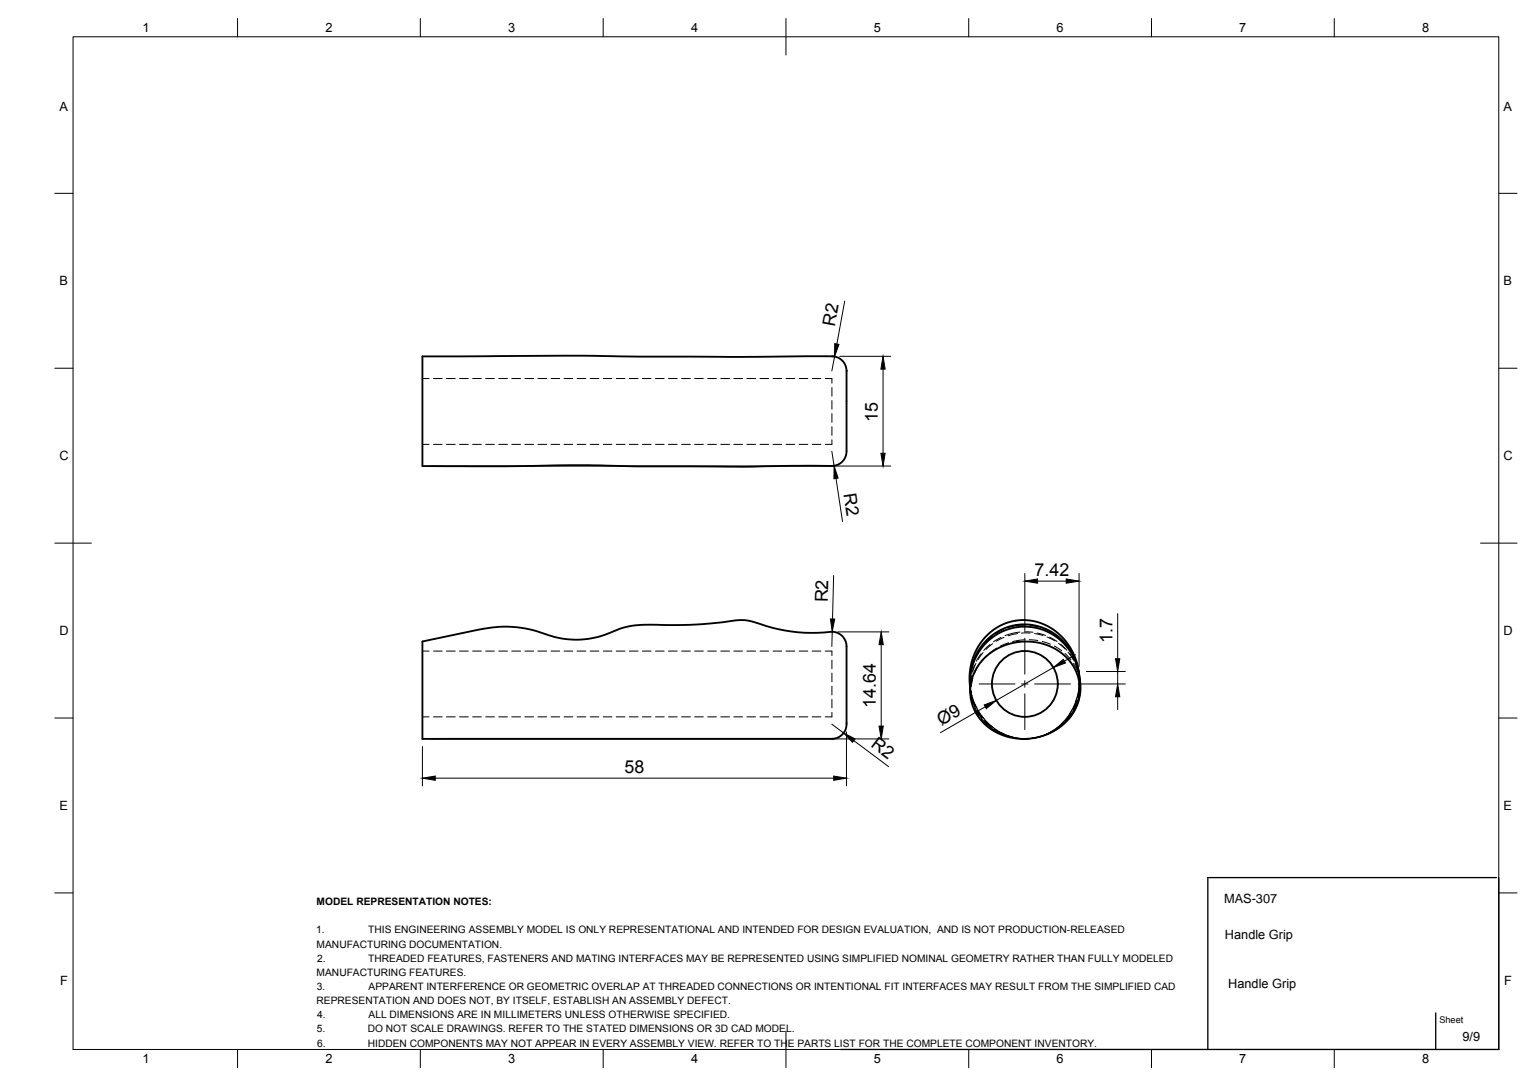
ISO-10303-21;
HEADER;
FILE_DESCRIPTION (('STEP AP214'),
    '1' );
FILE_NAME ('Handle Grip.step',
    '2026-10-06T07:34:29',
    ( '' ),
    ( '' ),
    'SwSTEP 2.0',
    'SolidWorks 2025',
    '' );
FILE_SCHEMA (( 'AUTOMOTIVE_DESIGN' ));
ENDSEC;

DATA;
#6=CARTESIAN_POINT ( 'NONE',  ( -167.5053995445195767, 127.4304153265770907, 2.500000001036336350 ) ) ;
#10=CARTESIAN_POINT ( 'NONE',  ( -168.3602667112202766, 125.8948777600411830, -3.002243219525047024 ) ) ;
#25=CARTESIAN_POINT ( 'NONE',  ( -225.5636091402884915, 143.1065995042388863, -0.5218507872395625746 ) ) ;
#28=CARTESIAN_POINT ( 'NONE',  ( -185.2335129678179726, 125.0353967269121966, 9.577123744044223841 ) ) ;
#58=FACE_OUTER_BOUND ( 'NONE', #1129, .T. ) ;
#68=CARTESIAN_POINT ( 'NONE',  ( -223.5763732829059904, 146.6670444861485976, 6.843617190574383891 ) ) ;
#87=CARTESIAN_POINT ( 'NONE',  ( -207.0700983879231387, 149.0508413170868209, -0.4547266291960758156 ) ) ;
#99=CARTESIAN_POINT ( 'NONE',  ( -218.1518098834511648, 139.2461763302102327, 3.478895870929506362 ) ) ;
#102=CARTESIAN_POINT ( 'NONE',  ( -182.6699909761611877, 123.4132960977408970, 9.577123744044220288 ) ) ;
#112=CARTESIAN_POINT ( 'NONE',  ( -225.3482675701515348, 143.4924177300907502, -0.7821592797845021705 ) ) ;
#133=CARTESIAN_POINT ( 'NONE',  ( -221.9693044472552117, 149.5463605724702916, 7.947916423171728084 ) ) ;
#136=CARTESIAN_POINT ( 'NONE',  ( -222.7380986314676363, 148.1689451111236906, 7.733218891984481758 ) ) ;
#137=EDGE_CURVE ( 'NONE', #9526, #14472, #1038, .T. ) ;
#142=CIRCLE ( 'NONE', #13010, 4.499999999999950262 ) ;
#146=B_SPLINE_CURVE_WITH_KNOTS ( 'NONE', 3,
 ( #5136, #531, #1653, #11218, #9963, #14979, #8698, #12464, #14906, #1729, #5371, #4019, #13643, #371, #7438, #2772, #5212, #6490, #11287, #14749, #7674, #6569, #448, #13727, #10034, #10112, #10189, #12233, #8933, #1411, #2930, #11372, #4170, #6248, #1492, #211, #11061, #2692, #5059, #9884, #14674, #3874, #685, #1881, #15369, #849, #13889, #9240 ),
 .UNSPECIFIED., .F., .F.,
 ( 4, 2, 2, 2, 2, 2, 2, 2, 2, 2, 2, 2, 2, 2, 2, 2, 2, 2, 2, 2, 2, 2, 2, 4 ),
 ( 0.02192817935270313656, 0.02330785662426448565, 0.02399769526004516540, 0.02468753389582584862, 0.02606721116738722893, 0.02675704980316793297, 0.02744688843894863700, 0.02882656571051007630, 0.02951640434629079768, 0.03020624298207151559, 0.03158592025363299305, 0.03227575888941371096, 0.03296559752519442887, 0.03365543616097514679, 0.03434527479675586470, 0.03572495206831733522, 0.03641479070409808783, 0.03710462933987884043, 0.03779446797565959304, 0.03848430661144034565, 0.03986398388300183004, 0.04124366115456330750, 0.04262333842612478496, 0.04400301569768626936 ),
 .UNSPECIFIED. ) ;
#156=CARTESIAN_POINT ( 'NONE',  ( -179.9223906590855222, 134.3711564447467310, 1.515441477536284554 ) ) ;
#157=CARTESIAN_POINT ( 'NONE',  ( -223.6137413416247739, 142.0138547493179146, 2.263321283727593336 ) ) ;
#159=CIRCLE ( 'NONE', #9018, 4.499999999999950262 ) ;
#170=CARTESIAN_POINT ( 'NONE',  ( -183.7136537759689929, 127.7093858820786068, -5.230826428279597096 ) ) ;
#173=CARTESIAN_POINT ( 'NONE',  ( -197.4591130885309553, 135.0981391493542105, 10.16010209732750802 ) ) ;
#189=ORIENTED_EDGE ( 'NONE', *, *, #8600, .F. ) ;
#199=CARTESIAN_POINT ( 'NONE',  ( -185.2055264765504887, 137.3096093875189467, 2.500000000000000000 ) ) ;
#206=CARTESIAN_POINT ( 'NONE',  ( -224.5476011597490356, 144.9269372877251669, 3.604463283145519448 ) ) ;
#209=CARTESIAN_POINT ( 'NONE',  ( -222.3356595723642215, 144.5667354790973604, 8.419022500423421818 ) ) ;
#211=CARTESIAN_POINT ( 'NONE',  ( -172.9645346626803359, 118.3395572346633173, -3.768257758897336274 ) ) ;
#254=CARTESIAN_POINT ( 'NONE',  ( -176.4863952559862526, 117.0241230567913959, -0.6469977504890583875 ) ) ;
#257=CARTESIAN_POINT ( 'NONE',  ( -171.9895241055258168, 125.0924944214600885, 9.516496325551347724 ) ) ;
#271=CARTESIAN_POINT ( 'NONE',  ( -218.6464950597879238, 155.4996951832063701, 5.432615396193927637 ) ) ;
#288=CARTESIAN_POINT ( 'NONE',  ( -167.5097532647548633, 127.4226149533560175, 3.478855110549762042 ) ) ;
#292=CARTESIAN_POINT ( 'NONE',  ( -221.1247960154559280, 151.0594299935001743, 7.622044586438916802 ) ) ;
#294=CARTESIAN_POINT ( 'NONE',  ( -220.5689849208904150, 152.0552528170083519, 9.261189829759533865 ) ) ;
#304=B_SPLINE_CURVE_WITH_KNOTS ( 'NONE', 3,
 ( #12178, #157, #5002, #3249, #8007 ),
 .UNSPECIFIED., .F., .F.,
 ( 4, 1, 4 ),
 ( 2.671544684753287039E-05, 0.0004182544953931666577, 0.0008097935439387997673 ),
 .UNSPECIFIED. ) ;
#316=CARTESIAN_POINT ( 'NONE',  ( -214.8715905313398480, 153.8675021612092451, 2.500000000000000000 ) ) ;
#328=CARTESIAN_POINT ( 'NONE',  ( -223.3178949021943538, 142.5860305806809833, -0.6404123112780930605 ) ) ;
#330=CARTESIAN_POINT ( 'NONE',  ( -207.1238489746795608, 137.1336079999123854, -4.642206099735007641 ) ) ;
#333=CARTESIAN_POINT ( 'NONE',  ( -199.4124801547868913, 127.6177204676982910, 1.515400478619089109 ) ) ;
#358=CARTESIAN_POINT ( 'NONE',  ( -218.4414990732828699, 155.8669776719573861, 2.805362964459314323 ) ) ;
#359=CARTESIAN_POINT ( 'NONE',  ( -218.6464950597879238, 155.4996951832063701, 5.432615396193927637 ) ) ;
#367=CARTESIAN_POINT ( 'NONE',  ( -220.9628981692495699, 151.3494953986536018, 7.483278023344910324 ) ) ;
#369=CARTESIAN_POINT ( 'NONE',  ( -219.7507648086670429, 149.4749995001899663, 9.873895959572530856 ) ) ;
#371=CARTESIAN_POINT ( 'NONE',  ( -168.7841562197520489, 125.8293614238909299, -3.029850393553606303 ) ) ;
#395=CARTESIAN_POINT ( 'NONE',  ( -187.5347606140533969, 120.9941390333424636, 2.431555724346869063 ) ) ;
#405=CARTESIAN_POINT ( 'NONE',  ( -217.9852252332578928, 152.6415593000486126, -3.308226381094188095 ) ) ;
#406=CARTESIAN_POINT ( 'NONE',  ( -195.7742941377835280, 134.4381891934308442, -5.230826428279600648 ) ) ;
#409=CARTESIAN_POINT ( 'NONE',  ( -199.2256335332332640, 127.9713659812714042, 5.434137442415931218 ) ) ;
#443=CARTESIAN_POINT ( 'NONE',  ( -224.5811800873043182, 144.8667753680073531, 1.831365460742872209 ) ) ;
#446=CARTESIAN_POINT ( 'NONE',  ( -218.2326813014511799, 152.2161514369302324, 8.572300711411607210 ) ) ;
#448=CARTESIAN_POINT ( 'NONE',  ( -170.5205985377005220, 122.7182524358224640, -5.056862372992222632 ) ) ;
#483=CARTESIAN_POINT ( 'NONE',  ( -221.4307639069678544, 146.2562371466928255, -4.592498632207916209 ) ) ;
#485=CARTESIAN_POINT ( 'NONE',  ( -176.9844935205031504, 127.5518652045528825, -4.662307221713766658 ) ) ;
#488=CARTESIAN_POINT ( 'NONE',  ( -173.0737465816261818, 117.4314230949052558, 7.694953281110847421 ) ) ;
#500=CARTESIAN_POINT ( 'NONE',  ( -198.5721217036497990, 144.7598446228703324, 3.478855109513426580 ) ) ;
#517=CARTESIAN_POINT ( 'NONE',  ( -219.4169908596040273, 154.1192310103966179, 2.706804888356528771 ) ) ;
#529=CARTESIAN_POINT ( 'NONE',  ( -219.5915661803683463, 153.8064519195449407, 4.439938623566930254 ) ) ;
#531=CARTESIAN_POINT ( 'NONE',  ( -167.7969933075935387, 127.5980187394608549, 2.035704077629012954 ) ) ;
#543=MECHANICAL_DESIGN_GEOMETRIC_PRESENTATION_REPRESENTATION('',(#10911),#10658);
#570=CARTESIAN_POINT ( 'NONE',  ( -202.8891874331996519, 144.7632710727894505, -2.963320117457099112 ) ) ;
#573=CARTESIAN_POINT ( 'NONE',  ( -186.4931015233695462, 122.8215886266871593, 7.918248976830652097 ) ) ;
#586=CARTESIAN_POINT ( 'NONE',  ( -182.6699909761611877, 123.4132960977408970, 9.577123744044220288 ) ) ;
#599=CARTESIAN_POINT ( 'NONE',  ( -169.3917585582371714, 124.7407464570165700, 8.854531459401838944 ) ) ;
#600=CARTESIAN_POINT ( 'NONE',  ( -219.0516113763855799, 154.7738657095153769, -1.749095451262919765 ) ) ;
#611=CARTESIAN_POINT ( 'NONE',  ( -220.4620190166787950, 152.2468990252863819, 9.155722436418765042 ) ) ;
#647=CARTESIAN_POINT ( 'NONE',  ( -187.0868153883506011, 133.8486679469899343, -4.640918829492425957 ) ) ;
#650=CARTESIAN_POINT ( 'NONE',  ( -214.6174474432871762, 135.6318802667844921, 5.434137442415934771 ) ) ;
#661=CARTESIAN_POINT ( 'NONE',  ( -191.1905365997726562, 133.0085349363843363, 10.16010209732750624 ) ) ;
#671=CARTESIAN_POINT ( 'NONE',  ( -169.9972604110092789, 123.6558948400181634, 9.476346162107795124 ) ) ;
#672=CARTESIAN_POINT ( 'NONE',  ( -218.9426345149119300, 150.9185095621452035, -4.524781484457172986 ) ) ;
#685=CARTESIAN_POINT ( 'NONE',  ( -173.9738588760758944, 116.5311944691898560, -0.9961046041182962663 ) ) ;
#700=CARTESIAN_POINT ( 'NONE',  ( -225.6985468192879409, 142.8648374703979016, 2.076118051499458161 ) ) ;
#713=APPLICATION_CONTEXT ( 'automotive_design' ) ;
#717=ADVANCED_FACE ( 'NONE', ( #1332, #7434 ), #1486, .F. ) ;
#722=CARTESIAN_POINT ( 'NONE',  ( -169.4320859569187405, 123.9702250307836238, -4.722862203412457660 ) ) ;
#725=CARTESIAN_POINT ( 'NONE',  ( -195.7742941377835280, 134.4381891934308442, -5.230826428279600648 ) ) ;
#742=CARTESIAN_POINT ( 'NONE',  ( -174.5069932933876942, 126.2863744793834826, 9.536681319450917016 ) ) ;
#756=CARTESIAN_POINT ( 'NONE',  ( -173.9115424460105430, 116.6428441356814432, 5.774694861875956597 ) ) ;
#757=CARTESIAN_POINT ( 'NONE',  ( -222.4281468042453298, 148.7242724638446703, -5.036090039102246507 ) ) ;
#765=EDGE_CURVE ( 'NONE', #9030, #14554, #2287, .T. ) ;
#766=CARTESIAN_POINT ( 'NONE',  ( -219.7707515679132655, 153.4854131703968392, -0.3598758019112536233 ) ) ;
#773=CARTESIAN_POINT ( 'NONE',  ( -170.1275826011421941, 128.8939672761866859, 2.500000000760459695 ) ) ;
#805=CARTESIAN_POINT ( 'NONE',  ( -170.8299300849453459, 127.1729693371208043, -2.992655347556774981 ) ) ;
#808=CARTESIAN_POINT ( 'NONE',  ( -219.6417540138374704, 145.3326194796887023, -4.642206099735023628 ) ) ;
#824=CARTESIAN_POINT ( 'NONE',  ( -216.9711578880983893, 150.1110767499728240, 9.578254705571840333 ) ) ;
#835=CARTESIAN_POINT ( 'NONE',  ( -168.4340493060770427, 126.4566329172550070, 6.894248570768724882 ) ) ;
#836=CARTESIAN_POINT ( 'NONE',  ( -222.5645123348796801, 148.4799522099133640, -2.927675643679180428 ) ) ;
#849=CARTESIAN_POINT ( 'NONE',  ( -174.2601771783465097, 116.0182102862799383, 1.243088744850515459 ) ) ;
#850=CARTESIAN_POINT ( 'NONE',  ( -216.7144175016715337, 154.8588128942135143, 3.150775860475527601 ) ) ;
#853=CARTESIAN_POINT ( 'NONE',  ( -210.7165899865938172, 151.5484195431892545, 2.500000000000000000 ) ) ;
#859=EDGE_CURVE ( 'NONE', #14554, #9030, #3433, .T. ) ;
#867=CARTESIAN_POINT ( 'NONE',  ( -223.5869895076567957, 142.0744606454175312, 3.511683908622253991 ) ) ;
#886=CARTESIAN_POINT ( 'NONE',  ( -191.3370974917540366, 126.0439545877573266, -0.4555467707853441128 ) ) ;
#897=SURFACE_STYLE_FILL_AREA ( #8426 ) ;
#901=CARTESIAN_POINT ( 'NONE',  ( -185.2335129678179726, 125.0353967269121966, 9.577123744044223841 ) ) ;
#914=CARTESIAN_POINT ( 'NONE',  ( -221.3664521364747202, 150.6264651190829511, -2.887957967080375443 ) ) ;
#964=CARTESIAN_POINT ( 'NONE',  ( -223.5232045190763301, 146.7623046726374980, -4.689260562946596878 ) ) ;
#978=CARTESIAN_POINT ( 'NONE',  ( -214.6152097961127367, 135.6358893629490581, -0.4555467707853336767 ) ) ;
#992=CARTESIAN_POINT ( 'NONE',  ( -222.3946175953714999, 148.7843453047176467, -2.994737441843033476 ) ) ;
#1000=CARTESIAN_POINT ( 'NONE',  ( -206.0179204244930702, 148.9258921110169638, 2.500000000000000000 ) ) ;
#1007=AXIS2_PLACEMENT_3D ( 'NONE', #2898, #5252, #7561 ) ;
#1011=CARTESIAN_POINT ( 'NONE',  ( -216.7032046242510148, 154.8780296845847033, 2.891444798692482721 ) ) ;
#1013=CARTESIAN_POINT ( 'NONE',  ( -193.7200834347810599, 142.0619459586758921, 2.500000000000000000 ) ) ;
#1038=CIRCLE ( 'NONE', #11412, 4.499999999999950262 ) ;
#1051=CARTESIAN_POINT ( 'NONE',  ( -181.1480734112017501, 126.1383063644306617, -5.230826428279600648 ) ) ;
#1053=EDGE_LOOP ( 'NONE', ( #1556, #9864 ) ) ;
#1066=CARTESIAN_POINT ( 'NONE',  ( -213.9961813491638623, 134.6717504882919911, 1.515400478619087776 ) ) ;
#1073=CARTESIAN_POINT ( 'NONE',  ( -217.6653619995784652, 138.6635820529667740, 2.431555724346871283 ) ) ;
#1078=CARTESIAN_POINT ( 'NONE',  ( -219.3877568461323619, 150.1024971847152756, -4.823803736792959818 ) ) ;
#1079=CARTESIAN_POINT ( 'NONE',  ( -223.4717893243274602, 142.3106348291761662, 4.713848895078025514 ) ) ;
#1089=ORIENTED_EDGE ( 'NONE', *, *, #5398, .F. ) ;
#1094=CARTESIAN_POINT ( 'NONE',  ( -218.4488137430494419, 155.8538722928748541, 3.478855109783925315 ) ) ;
#1105=CARTESIAN_POINT ( 'NONE',  ( -224.7518895393548348, 144.5609225879004498, 7.521475632127809341 ) ) ;
#1111=CYLINDRICAL_SURFACE ( 'NONE', #6828, 4.499999999999950262 ) ;
#1127=CARTESIAN_POINT ( 'NONE',  ( -216.9311889273521672, 150.1826874172201656, -4.640918829492440167 ) ) ;
#1129=EDGE_LOOP ( 'NONE', ( #6452, #6459, #7636, #5771, #1089 ) ) ;
#1140=CARTESIAN_POINT ( 'NONE',  ( -225.7548303624724610, 142.7639966680278576, 1.446957622915672204 ) ) ;
#1144=CARTESIAN_POINT ( 'NONE',  ( -203.7296541848517109, 135.3294987143146955, 9.577123744044227394 ) ) ;
#1155=CARTESIAN_POINT ( 'NONE',  ( -218.9545055651059045, 150.9247396209540568, 9.391049919365073606 ) ) ;
#1176=CARTESIAN_POINT ( 'NONE',  ( -224.5448265106511769, 144.9319085071302879, 3.590746859383691536 ) ) ;
#1194=CARTESIAN_POINT ( 'NONE',  ( -202.8891874331996519, 144.7632710727894505, -2.963320117457099112 ) ) ;
#1212=CARTESIAN_POINT ( 'NONE',  ( -191.4964613557999655, 125.7493975051623352, 3.478895870929489043 ) ) ;
#1215=CARTESIAN_POINT ( 'NONE',  ( -210.0240857098682454, 141.7683007401625446, 10.16010209732750624 ) ) ;
#1228=CARTESIAN_POINT ( 'NONE',  ( -224.5811800873044604, 144.8667753680074384, 1.831365460742872209 ) ) ;
#1258=CARTESIAN_POINT ( 'NONE',  ( -221.2417723974670878, 146.6801937162670697, 9.651042165284529517 ) ) ;
#1280=CARTESIAN_POINT ( 'NONE',  ( -178.3861577417919477, 131.0834419243807076, -2.963320117457100888 ) ) ;
#1295=CARTESIAN_POINT ( 'NONE',  ( -200.9709139173866959, 128.5579952147370761, 5.434137442415933883 ) ) ;
#1298=CARTESIAN_POINT ( 'NONE',  ( -216.9711578880983893, 150.1110767499728240, 9.578254705571840333 ) ) ;
#1308=CARTESIAN_POINT ( 'NONE',  ( -225.6439726407676005, 142.9626156777225390, 1.090105839479173833 ) ) ;
#1316=CARTESIAN_POINT ( 'NONE',  ( -198.5677679834141713, 144.7676449960911498, 2.500000000000000000 ) ) ;
#1332=FACE_BOUND ( 'NONE', #3235, .T. ) ;
#1335=CARTESIAN_POINT ( 'NONE',  ( -224.2877105866247973, 145.3925720454151929, 5.086385912607861215 ) ) ;
#1342=CARTESIAN_POINT ( 'NONE',  ( -220.3531759299249302, 148.3382346779569616, 2.431557144026069928 ) ) ;
#1355=CARTESIAN_POINT ( 'NONE',  ( -188.7806045336324132, 137.2844789098840863, -2.963320117457101777 ) ) ;
#1369=CARTESIAN_POINT ( 'NONE',  ( -216.7159361415700403, 154.8568568287998630, 1.560284994380096046 ) ) ;
#1370=CARTESIAN_POINT ( 'NONE',  ( -183.9200705329474772, 121.1751083001002485, -2.964974570226829087 ) ) ;
#1373=CARTESIAN_POINT ( 'NONE',  ( -212.4168668197547731, 139.5435760318306677, 9.577123744044230946 ) ) ;
#1378=EDGE_CURVE ( 'NONE', #4070, #14472, #12986, .T. ) ;
#1385=CARTESIAN_POINT ( 'NONE',  ( -169.9361637590235716, 128.7768979049109532, 3.478855110294483133 ) ) ;
#1407=CARTESIAN_POINT ( 'NONE',  ( -221.6235305807591658, 150.1658687316387670, 7.893372954062758851 ) ) ;
#1409=CARTESIAN_POINT ( 'NONE',  ( -224.3998921539632931, 145.1915811579927151, 4.610672262717653069 ) ) ;
#1411=CARTESIAN_POINT ( 'NONE',  ( -171.8695707977107645, 120.3013568790891554, -4.955367435459418601 ) ) ;
#1432=CARTESIAN_POINT ( 'NONE',  ( -195.9617019660094570, 137.8802668252396586, -4.640918829492428621 ) ) ;
#1442=CARTESIAN_POINT ( 'NONE',  ( -217.5100339609262221, 153.4805093641580527, -2.286312808770087912 ) ) ;
#1444=CARTESIAN_POINT ( 'NONE',  ( -205.6342130761154863, 139.8173426991758959, -5.230826428279590878 ) ) ;
#1448=CARTESIAN_POINT ( 'NONE',  ( -181.1823003367078115, 126.0769834546670296, 10.16010209732750624 ) ) ;
#1451=ORIENTED_EDGE ( 'NONE', *, *, #9650, .T. ) ;
#1460=CARTESIAN_POINT ( 'NONE',  ( -186.0759242617834559, 135.7072545306847076, 7.919662025281895446 ) ) ;
#1477=CARTESIAN_POINT ( 'NONE',  ( -206.2408270422487249, 148.5277750773568926, 5.434754235172608361 ) ) ;
#1486=PLANE ( 'NONE',  #8630 ) ;
#1490=CARTESIAN_POINT ( 'NONE',  ( -219.4551987602064855, 154.0507755588392911, 3.411546396426036409 ) ) ;
#1492=CARTESIAN_POINT ( 'NONE',  ( -172.7841977562675311, 118.6626591106209787, -4.047107877712195823 ) ) ;
#1530=CARTESIAN_POINT ( 'NONE',  ( -220.2566479300740241, 148.4875731452288221, -5.069746451151177169 ) ) ;
#1531=CARTESIAN_POINT ( 'NONE',  ( -212.3935931674892856, 139.5852744332111683, -4.642206099735020963 ) ) ;
#1534=CARTESIAN_POINT ( 'NONE',  ( -217.9748787080196450, 139.5740753954225966, -0.4555467707853197989 ) ) ;
#1549=CARTESIAN_POINT ( 'NONE',  ( -218.4488137430494419, 155.8538722928748541, 3.478855109783925315 ) ) ;
#1556=ORIENTED_EDGE ( 'NONE', *, *, #3132, .T. ) ;
#1564=CARTESIAN_POINT ( 'NONE',  ( -185.3757041553864156, 136.9956776582455973, 5.434754235172603920 ) ) ;
#1571=CARTESIAN_POINT ( 'NONE',  ( -221.8318359980363539, 149.7926568781921048, 9.921711862944807336 ) ) ;
#1594=CARTESIAN_POINT ( 'NONE',  ( -169.9274309510963406, 128.7925441011331031, 1.515441478317341994 ) ) ;
#1612=CARTESIAN_POINT ( 'NONE',  ( -216.6980668629938123, 154.8869363267023687, 2.500000000158653091 ) ) ;
#1614=CARTESIAN_POINT ( 'NONE',  ( -202.2493014528935475, 138.0335512477381883, -5.230826428279597096 ) ) ;
#1617=CARTESIAN_POINT ( 'NONE',  ( -194.2694872093395873, 127.5478817636406035, 5.434137442415935659 ) ) ;
#1629=CARTESIAN_POINT ( 'NONE',  ( -169.2610106913410277, 124.9750017845142764, 2.431557144026069928 ) ) ;
#1643=CARTESIAN_POINT ( 'NONE',  ( -207.0940556909077657, 149.0079180481279479, 5.434754235172608361 ) ) ;
#1649=CARTESIAN_POINT ( 'NONE',  ( -224.5619881126438315, 144.9011608032434992, 1.476503984934130598 ) ) ;
#1651=CARTESIAN_POINT ( 'NONE',  ( -220.7901307343587689, 151.6590353782033560, 9.451677507526856203 ) ) ;
#1653=CARTESIAN_POINT ( 'NONE',  ( -167.8131253141077650, 127.5691157174926644, 1.575245659892765326 ) ) ;
#1686=CARTESIAN_POINT ( 'NONE',  ( -223.4327756907198648, 142.3614043895485963, 0.01469651188060598634 ) ) ;
#1687=CARTESIAN_POINT ( 'NONE',  ( -182.6467173238959560, 123.4549944991208292, -4.642206099735001423 ) ) ;
#1690=CARTESIAN_POINT ( 'NONE',  ( -194.4337897068680547, 127.2572260587109554, 3.478895870929501033 ) ) ;
#1716=CARTESIAN_POINT ( 'NONE',  ( -219.5038107907490144, 153.9636794753398874, -2.869066018171615884 ) ) ;
#1721=PRODUCT_DEFINITION_FORMATION_WITH_SPECIFIED_SOURCE ( 'ANY', '', #8040, .NOT_KNOWN. ) ;
#1725=CARTESIAN_POINT ( 'NONE',  ( -223.5023877966752366, 146.7996010984935538, -2.058674290867560153 ) ) ;
#1727=CARTESIAN_POINT ( 'NONE',  ( -219.7785425680613400, 153.4714543706508891, 5.235913750827374535 ) ) ;
#1729=CARTESIAN_POINT ( 'NONE',  ( -168.3225553318488892, 126.6563918736861325, -1.708925576422542392 ) ) ;
#1731=VERTEX_POINT ( 'NONE', #11313 ) ;
#1767=CARTESIAN_POINT ( 'NONE',  ( -194.3489852843322581, 137.1051365066642234, -4.640918829492427733 ) ) ;
#1770=CARTESIAN_POINT ( 'NONE',  ( -205.9652191273047777, 131.2378527988410326, 1.515400478619091329 ) ) ;
#1782=CARTESIAN_POINT ( 'NONE',  ( -204.9546745879972889, 133.0893851581147374, 7.918248976830629893 ) ) ;
#1793=CARTESIAN_POINT ( 'NONE',  ( -174.2824251065520968, 115.9783496305641535, 2.177446462082195389 ) ) ;
#1794=CARTESIAN_POINT ( 'NONE',  ( -217.7719644788709559, 153.0191138716839134, -2.888063911326615774 ) ) ;
#1806=CARTESIAN_POINT ( 'NONE',  ( -221.2434695521093602, 150.8468077239669753, 9.749916661835451137 ) ) ;
#1840=CARTESIAN_POINT ( 'NONE',  ( -218.4400809351218413, 155.8695184890967482, 1.515441477806783510 ) ) ;
#1843=CARTESIAN_POINT ( 'NONE',  ( -213.9961813491638623, 134.6717504882919911, 1.515400478619087776 ) ) ;
#1856=CARTESIAN_POINT ( 'NONE',  ( -218.3193879687431433, 147.6986783750013217, 10.16010209732750980 ) ) ;
#1868=CARTESIAN_POINT ( 'NONE',  ( -167.8057708040753653, 127.5822924766788447, 2.966601681492425868 ) ) ;
#1869=CARTESIAN_POINT ( 'NONE',  ( -217.8572871788818475, 152.8680898606328356, -3.058345895658412417 ) ) ;
#1881=CARTESIAN_POINT ( 'NONE',  ( -174.1255661870616507, 116.2593870075281473, -0.1232875569927439491 ) ) ;
#1917=CARTESIAN_POINT ( 'NONE',  ( -174.7802519396333878, 131.5011100042426904, 1.515441477806783066 ) ) ;
#1919=ORIENTED_EDGE ( 'NONE', *, *, #7073, .F. ) ;
#1920=CARTESIAN_POINT ( 'NONE',  ( -178.4115273750087738, 119.2860570028907858, -3.078262048313290311 ) ) ;
#1932=CARTESIAN_POINT ( 'NONE',  ( -170.7405378081422214, 121.6209906574826931, 10.02899269843361374 ) ) ;
#1942=CARTESIAN_POINT ( 'NONE',  ( -173.2932605743736474, 117.7505931626010778, 7.695635371731032848 ) ) ;
#1943=CARTESIAN_POINT ( 'NONE',  ( -222.5489981585923545, 148.5077482920355862, -5.007338236124175168 ) ) ;
#1962=ADVANCED_FACE ( 'NONE', ( #8477 ), #1111, .F. ) ;
#1995=CARTESIAN_POINT ( 'NONE',  ( -206.0135413368010404, 148.9337379340180405, 1.515441477536285220 ) ) ;
#1998=CARTESIAN_POINT ( 'NONE',  ( -190.6388552492889517, 127.3288340616119143, -2.964974570226841522 ) ) ;
#2013=CARTESIAN_POINT ( 'NONE',  ( -216.0863581598438543, 143.0557482234525253, 9.577123744044239828 ) ) ;
#2029=CARTESIAN_POINT ( 'NONE',  ( -224.6670067989573454, 144.7130033415326977, -2.813789935910935736 ) ) ;
#2076=CARTESIAN_POINT ( 'NONE',  ( -199.5653198453618700, 142.9393910578133102, -2.963320117457100000 ) ) ;
#2079=CARTESIAN_POINT ( 'NONE',  ( -183.9200705329474772, 121.1751083001002485, -2.964974570226829087 ) ) ;
#2098=CARTESIAN_POINT ( 'NONE',  ( -212.4168668197547731, 139.5435760318306677, 9.577123744044230946 ) ) ;
#2108=CARTESIAN_POINT ( 'NONE',  ( -171.9943068686860386, 120.0778726276766122, 9.490183841837444234 ) ) ;
#2109=CARTESIAN_POINT ( 'NONE',  ( -221.8782673190587786, 149.7094678780528909, -3.059957786404165603 ) ) ;
#2112=CARTESIAN_POINT ( 'NONE',  ( -218.3504703772591711, 152.0071873827878335, 8.737647451593067771 ) ) ;
#2125=CARTESIAN_POINT ( 'NONE',  ( -179.9267697467775520, 134.3633106217456543, 2.500000000000000000 ) ) ;
#2156=CARTESIAN_POINT ( 'NONE',  ( -181.0860728093183809, 120.2032420692993071, -3.023257939496618807 ) ) ;
#2173=CARTESIAN_POINT ( 'NONE',  ( -214.8265656857867327, 135.2606554265309740, 3.478895870929493483 ) ) ;
#2177=CARTESIAN_POINT ( 'NONE',  ( -218.1600191662880661, 152.2676192875508718, 2.431557144026069928 ) ) ;
#2186=CARTESIAN_POINT ( 'NONE',  ( -222.7845331223101084, 143.6298233191951113, -2.509092009812623925 ) ) ;
#2187=CARTESIAN_POINT ( 'NONE',  ( -223.5258475410019230, 142.2005172455266973, 4.260778343889476183 ) ) ;
#2215=FACE_OUTER_BOUND ( 'NONE', #12535, .T. ) ;
#2231=CARTESIAN_POINT ( 'NONE',  ( -167.5010204568278027, 127.4382611495783237, 1.515441478572621570 ) ) ;
#2235=CARTESIAN_POINT ( 'NONE',  ( -183.7136537759689929, 127.7093858820786068, -5.230826428279597096 ) ) ;
#2251=CARTESIAN_POINT ( 'NONE',  ( -175.7482920159357604, 118.3486081613139334, 7.749957389927518925 ) ) ;
#2266=CARTESIAN_POINT ( 'NONE',  ( -225.1194665507443915, 143.9023506720278647, -1.657832751462523291 ) ) ;
#2268=CARTESIAN_POINT ( 'NONE',  ( -222.8945441032406052, 143.4659034320898172, 7.188384078066360594 ) ) ;
#2282=CARTESIAN_POINT ( 'NONE',  ( -185.2055264765504887, 137.3096093875189467, 2.500000000000000000 ) ) ;
#2287=B_SPLINE_CURVE_WITH_KNOTS ( 'NONE', 3,
 ( #9719, #2846, #12229, #14514, #206, #5055, #2688, #11138, #13559, #6405, #11214, #6171, #2763, #14745, #13639, #14817, #3943, #3869, #7668, #133, #9880, #1407, #6240, #292, #367, #14590, #8764, #8694, #6092, #3792, #8614, #13411, #5208, #13484, #14670, #2609, #7590, #7507 ),
 .UNSPECIFIED., .F., .F.,
 ( 4, 2, 2, 2, 2, 2, 2, 2, 2, 2, 2, 2, 2, 2, 2, 2, 2, 2, 4 ),
 ( 0.03344994383916276293, 0.03451359215648128198, 0.03557724047379980103, 0.03664088879111832009, 0.03770453710843683914, 0.03876818542575535820, 0.03983183374307387725, 0.04089548206039239631, 0.04195913037771091536, 0.04249095453637018877, 0.04302277869502946217, 0.04408642701234789796, 0.04515007532966634068, 0.04621372364698477647, 0.04727737196430321920, 0.04780919612296243015, 0.04834102028162165499, 0.04940466859894009077, 0.05046831691625852656 ),
 .UNSPECIFIED. ) ;
#2295=CARTESIAN_POINT ( 'NONE',  ( -223.0729251748932427, 143.1115555702249083, 6.635881932953087592 ) ) ;
#2315=CARTESIAN_POINT ( 'NONE',  ( -211.2987210398670186, 151.8733316563206586, 2.500000000000000000 ) ) ;
#2319=CARTESIAN_POINT ( 'NONE',  ( -214.8672114436478466, 153.8753479842104355, 1.515441477536284998 ) ) ;
#2330=( NAMED_UNIT ( * ) PLANE_ANGLE_UNIT ( ) SI_UNIT ( $, .RADIAN. ) );
#2336=CARTESIAN_POINT ( 'NONE',  ( -182.0950013669840359, 118.3955881831737997, 3.410453015226076801 ) ) ;
#2339=CARTESIAN_POINT ( 'NONE',  ( -170.8670245162619779, 127.1065088405712373, 7.890326795182211583 ) ) ;
#2348=CARTESIAN_POINT ( 'NONE',  ( -224.5619895614427435, 144.9011582074930971, 1.476530791908167606 ) ) ;
#2349=CARTESIAN_POINT ( 'NONE',  ( -219.6010272286711142, 149.7497771715804618, 9.815441629410450730 ) ) ;
#2364=CARTESIAN_POINT ( 'NONE',  ( -177.3557003870508595, 132.9282874014947140, 2.500000000000000000 ) ) ;
#2376=CARTESIAN_POINT ( 'NONE',  ( -224.2465401054903964, 145.4663354250427574, 5.241715744539080291 ) ) ;
#2396=CARTESIAN_POINT ( 'NONE',  ( -187.9088347589046748, 138.8287307560422903, 1.515441477536284109 ) ) ;
#2410=CARTESIAN_POINT ( 'NONE',  ( -176.4886329031608909, 117.0201139606268441, 5.242686462712208062 ) ) ;
#2413=CARTESIAN_POINT ( 'NONE',  ( -189.9062345257129323, 135.2872556402745374, 9.578254705571842109 ) ) ;
#2426=CARTESIAN_POINT ( 'NONE',  ( -222.6177564301690950, 144.0132851167816170, 7.888750748740434027 ) ) ;
#2430=CARTESIAN_POINT ( 'NONE',  ( -206.8718859864436581, 149.4025266312245037, 2.500000000000000000 ) ) ;
#2449=CARTESIAN_POINT ( 'NONE',  ( -224.4594852000661831, 145.0848108613691920, 4.280488621519050518 ) ) ;
#2465=CARTESIAN_POINT ( 'NONE',  ( -174.7846310273254176, 131.4932641812416421, 2.500000000270498735 ) ) ;
#2469=CARTESIAN_POINT ( 'NONE',  ( -204.1471980322648960, 142.4963817258166614, -4.640918829492428621 ) ) ;
#2488=CARTESIAN_POINT ( 'NONE',  ( -205.7712766299887335, 131.5939592662764994, -0.4555467707853333992 ) ) ;
#2491=CARTESIAN_POINT ( 'NONE',  ( -173.3366878899875019, 128.3846004176512849, 7.899914667150486736 ) ) ;
#2501=CARTESIAN_POINT ( 'NONE',  ( -223.5232359142329699, 142.1851836626728129, 0.6707363232510722417 ) ) ;
#2523=CARTESIAN_POINT ( 'NONE',  ( -198.5721217036497990, 144.7598446228703324, 3.478855109513426580 ) ) ;
#2532=CARTESIAN_POINT ( 'NONE',  ( -222.5506325035290729, 148.5048201065549733, 9.875490118357738822 ) ) ;
#2557=CARTESIAN_POINT ( 'NONE',  ( -174.4670243326416994, 126.3579851466298010, -4.682492215613329734 ) ) ;
#2569=CARTESIAN_POINT ( 'NONE',  ( -221.1246142512582082, 146.8432591943234797, -4.818913680500031660 ) ) ;
#2570=CARTESIAN_POINT ( 'NONE',  ( -175.7369819406991382, 118.3688719364822646, -3.133266157129962259 ) ) ;
#2576=CARTESIAN_POINT ( 'NONE',  ( -213.7333075327791789, 137.2030432634720967, 7.918248976830621011 ) ) ;
#2578=CARTESIAN_POINT ( 'NONE',  ( -173.6473242186147274, 117.1162325653264418, 2.431557144026069928 ) ) ;
#2596=ORIENTED_EDGE ( 'NONE', *, *, #137, .F. ) ;
#2609=CARTESIAN_POINT ( 'NONE',  ( -219.4906341098210589, 153.9872875675930857, 3.763523804975331011 ) ) ;
#2612=CARTESIAN_POINT ( 'NONE',  ( -223.5303683316520562, 142.1912745150580122, 4.217707172678373695 ) ) ;
#2634=CARTESIAN_POINT ( 'NONE',  ( -212.2154691228631691, 150.1790628786027355, -2.963320117457098224 ) ) ;
#2648=CARTESIAN_POINT ( 'NONE',  ( -219.5968554534879331, 149.7166363036416215, -4.923873429609202823 ) ) ;
#2649=CARTESIAN_POINT ( 'NONE',  ( -197.4248861630254055, 135.1594620591177431, -5.230826428279599760 ) ) ;
#2652=CARTESIAN_POINT ( 'NONE',  ( -224.7572118800429735, 144.5513867789856022, 7.859965607560822853 ) ) ;
#2667=CARTESIAN_POINT ( 'NONE',  ( -206.2408270422487249, 148.5277750773568926, 5.434754235172608361 ) ) ;
#2680=CARTESIAN_POINT ( 'NONE',  ( -207.1387806695930749, 146.9236570583465209, 7.919662025281895446 ) ) ;
#2684=EDGE_CURVE ( 'NONE', #8499, #4070, #159, .T. ) ;
#2688=CARTESIAN_POINT ( 'NONE',  ( -224.3981447419311905, 145.1947119209457355, 4.619413130059836448 ) ) ;
#2690=CARTESIAN_POINT ( 'NONE',  ( -217.0312179575220171, 154.3153628681492364, 5.590069521792075058 ) ) ;
#2692=CARTESIAN_POINT ( 'NONE',  ( -173.2167472191050592, 117.8876788491354546, -3.302252044790073615 ) ) ;
#2723=CARTESIAN_POINT ( 'NONE',  ( -216.8640855513551458, 154.6031491089179610, 0.1911473656376749541 ) ) ;
#2725=CARTESIAN_POINT ( 'NONE',  ( -179.1950877003932874, 117.8811570380880909, -0.5844242688643165318 ) ) ;
#2728=EDGE_CURVE ( 'NONE', #4058, #9509, #5255, .T. ) ;
#2729=CARTESIAN_POINT ( 'NONE',  ( -209.4369489341841586, 132.9646294043573675, 1.515400478619103763 ) ) ;
#2742=CARTESIAN_POINT ( 'NONE',  ( -175.8063512637129975, 129.6626919947313468, 7.909502539118761888 ) ) ;
#2758=CARTESIAN_POINT ( 'NONE',  ( -215.0595991585972513, 153.5311831015895052, 5.434754235172610137 ) ) ;
#2763=CARTESIAN_POINT ( 'NONE',  ( -223.4350041415068802, 146.9203294941767979, 7.065198963530563425 ) ) ;
#2768=CARTESIAN_POINT ( 'NONE',  ( -217.3957880433649450, 153.6844344254827490, 6.840999781109323052 ) ) ;
#2772=CARTESIAN_POINT ( 'NONE',  ( -169.1985897318295144, 125.0868387319165862, -3.803836676538010497 ) ) ;
#2808=CARTESIAN_POINT ( 'NONE',  ( -217.5843001957448450, 153.3500559703123827, -2.470211307036358495 ) ) ;
#2809=CARTESIAN_POINT ( 'NONE',  ( -211.5558396979514839, 139.0314540006070274, -4.642206099735020963 ) ) ;
#2812=CARTESIAN_POINT ( 'NONE',  ( -193.5534063424729254, 128.8169105028637205, 7.918248976830644992 ) ) ;
#2825=CARTESIAN_POINT ( 'NONE',  ( -188.0905678060899220, 138.5068454852687125, 5.434754235172603920 ) ) ;
#2838=CARTESIAN_POINT ( 'NONE',  ( -220.0166125838651681, 153.0449145666497657, -1.086335426908857871 ) ) ;
#2839=CARTESIAN_POINT ( 'NONE',  ( -202.9262818645171649, 144.6968105762408072, 7.919662025281898998 ) ) ;
#2846=CARTESIAN_POINT ( 'NONE',  ( -224.6003591769690502, 144.8324130182638783, 2.185988691727169808 ) ) ;
#2848=CARTESIAN_POINT ( 'NONE',  ( -221.9533209457892156, 149.5749975243766130, 9.934841322514504469 ) ) ;
#2878=CARTESIAN_POINT ( 'NONE',  ( -222.5463326935617658, 144.4088500683630514, 2.431557144026069928 ) ) ;
#2886=CARTESIAN_POINT ( 'NONE',  ( -216.6959657076304211, 154.8907008763735291, 2.027593286600615219 ) ) ;
#2888=CARTESIAN_POINT ( 'NONE',  ( -213.7219974575431252, 137.2233070386400584, -2.964974570226852180 ) ) ;
#2891=CARTESIAN_POINT ( 'NONE',  ( -225.7548303624724610, 142.7639966680278576, 1.446957622915672204 ) ) ;
#2898=CARTESIAN_POINT ( 'NONE',  ( -171.4541674549778918, 121.0456171749203662, 2.431557144026069928 ) ) ;
#2904=CARTESIAN_POINT ( 'NONE',  ( -192.1748460459477030, 141.1892528453990110, 3.478855109513427468 ) ) ;
#2918=CARTESIAN_POINT ( 'NONE',  ( -216.7216729069046437, 154.8463875879167801, 3.280095325655319805 ) ) ;
#2925=CARTESIAN_POINT ( 'NONE',  ( -224.3577192346544109, 145.2671405629664605, 0.1302923617619599905 ) ) ;
#2927=CARTESIAN_POINT ( 'NONE',  ( -219.9692141781003443, 153.1298362508722448, 5.829181591414630326 ) ) ;
#2930=CARTESIAN_POINT ( 'NONE',  ( -172.0842878089050600, 119.9166576486493057, -4.812951232078420460 ) ) ;
#2961=CARTESIAN_POINT ( 'NONE',  ( -214.8672114436478466, 153.8753479842104355, 1.515441477536284998 ) ) ;
#2963=CARTESIAN_POINT ( 'NONE',  ( -179.1973253475678121, 117.8771479419235675, 5.305259944336949474 ) ) ;
#2976=CARTESIAN_POINT ( 'NONE',  ( -213.7333075327791789, 137.2030432634720967, 7.918248976830621011 ) ) ;
#2979=B_SPLINE_SURFACE_WITH_KNOTS ( 'NONE', 3, 3, ( 
 ( #10821, #12000, #7118, #10979, #8387, #3703, #13322, #3627, #6236, #11048, #199, #13167, #2364, #5047, #8461, #9552, #5999 ),
 ( #1094, #5917, #4897, #14505, #10738, #4814, #2523, #7354, #12149, #6162, #4970, #9787, #12295, #14741, #10026, #9949, #288 ),
 ( #359, #2758, #3936, #1643, #1477, #5201, #14810, #13634, #12455, #12378, #1564, #7582, #14666, #8758, #13552, #4006, #8840 ),
 ( #11207, #5126, #6400, #3864, #2680, #2839, #7660, #6476, #8687, #13479, #7502, #6318, #11132, #13215, #2491, #2339, #3909 ),
 ( #5097, #1298, #14402, #3600, #13292, #4867, #6056, #13137, #5021, #2413, #13375, #7403, #3673, #8659, #11103, #257, #7248 ),
 ( #9921, #8507, #11974, #12042, #1215, #8583, #6131, #173, #8436, #13453, #9762, #7473, #1448, #12193, #12269, #7324, #12121 ),
 ( #11023, #6285, #7171, #1373, #3754, #15578, #1144, #10952, #4943, #9685, #10874, #28, #102, #4782, #14478, #6211, #9847 ),
 ( #2652, #14551, #9606, #2576, #5970, #14640, #3837, #14713, #10789, #2812, #14864, #573, #7790, #10001, #5411, #11181, #488 ),
 ( #13526, #15095, #11490, #650, #12500, #14783, #3977, #8895, #409, #1617, #8732, #10227, #13606, #8973, #2963, #4059, #4208 ),
 ( #5490, #7633, #8809, #10304, #13685, #7552, #12425, #6448, #4134, #1690, #11408, #11254, #9045, #5327, #3044, #12656, #12573 ),
 ( #2891, #7714, #15021, #6605, #1843, #2729, #1770, #14944, #333, #12350, #6527, #10151, #5246, #10071, #11327, #13766, #5174 ),
 ( #13845, #7873, #1534, #6687, #6370, #11795, #10461, #12731, #14075, #3269, #886, #3117, #8110, #12893, #13928, #4445, #9127 ),
 ( #11723, #10380, #5569, #10693, #3425, #14228, #6912, #5718, #5875, #7948, #1998, #14154, #2079, #2156, #1920, #6991, #15173 ),
 ( #964, #808, #12809, #7069, #8185, #10528, #5642, #4288, #4368, #3349, #5791, #8259, #11879, #15326, #4525, #9355, #6755 ),
 ( #12969, #10616, #15406, #15249, #4606, #8021, #9429, #11562, #725, #9278, #13034, #2235, #1051, #9204, #3191, #14001, #6836 ),
 ( #11646, #1127, #6267, #14618, #9824, #2469, #7303, #1432, #14300, #13193, #9744, #9666, #13354, #8335, #2557, #10770, #6033 ),
 ( #12025, #8417, #2634, #3733, #13273, #1194, #15484, #15556, #14536, #1355, #3818, #7456, #1280, #6113, #12101, #4679, #10 ),
 ( #8560, #7384, #10855, #87, #3581, #10932, #9507, #13120, #4848, #4927, #12177, #6194, #11006, #14384, #14461, #8638, #4761 ),
 ( #3499, #2319, #12252, #7149, #3655, #5948, #9584, #8491, #7231, #2396, #11955, #156, #5001, #13435, #5307, #1594, #6590 ),
 ( #13823, #316, #11162, #7854, #6430, #9903, #9983, #5156, #6507, #4040, #13744, #12330, #11390, #7693, #5392, #15002, #10134 ) ),
 .UNSPECIFIED., .T., .F., .F.,
 ( 4, 1, 1, 1, 1, 1, 1, 1, 2, 1, 1, 1, 1, 1, 1, 1, 4 ),
 ( 4, 2, 2, 2, 2, 2, 3, 4 ),
 ( 0.000000000000000000, 0.06231844716590150685, 0.1246368943318030137, 0.1869553414977045136, 0.2492737886636060274, 0.3115922358295075134, 0.3739106829954090272, 0.4362291301613105410, 0.4985475773272120548, 0.5612291301613105965, 0.6239106829954090827, 0.6865922358295075689, 0.7492737886636060551, 0.8119553414977045414, 0.8746368943318030276, 0.9373184471659015138, 1.000000000000000000 ),
 ( 0.000000000000000000, 0.2455027589669699362, 0.3041813370740077405, 0.5308033955276700855, 0.6372805264318514018, 0.8233339832829627003, 1.000000000000000000, 1.166726064904226812 ),
 .UNSPECIFIED. ) ;
#2989=CARTESIAN_POINT ( 'NONE',  ( -172.2044971521971490, 119.7012837404576260, 9.318491256855141458 ) ) ;
#2990=CARTESIAN_POINT ( 'NONE',  ( -218.5136094644957723, 155.7377805866632627, 0.8972885290472901731 ) ) ;
#2998=CARTESIAN_POINT ( 'NONE',  ( -220.1893657699865230, 152.7354001160375674, -1.484330510406285830 ) ) ;
#3000=CARTESIAN_POINT ( 'NONE',  ( -219.4227507837628366, 154.1089112020831635, 7.576492947193309568 ) ) ;
#3040=CARTESIAN_POINT ( 'NONE',  ( -177.5434268683390826, 132.5922366007948199, -0.4547266291960713747 ) ) ;
#3044=CARTESIAN_POINT ( 'NONE',  ( -179.3772030532177837, 117.5545944912402661, 3.345861034185851235 ) ) ;
#3057=CARTESIAN_POINT ( 'NONE',  ( -193.5534063424729254, 128.8169105028637205, 7.918248976830644992 ) ) ;
#3064=VERTEX_POINT ( 'NONE', #14868 ) ;
#3069=CARTESIAN_POINT ( 'NONE',  ( -169.6864937364892683, 124.2126821195596165, 9.200833310921806785 ) ) ;
#3070=CARTESIAN_POINT ( 'NONE',  ( -216.6950415564453465, 154.8919953347533749, 2.805421358301762869 ) ) ;
#3079=CARTESIAN_POINT ( 'NONE',  ( -220.0166125836030915, 153.0449145671193492, -1.086335427222236527 ) ) ;
#3114=CARTESIAN_POINT ( 'NONE',  ( -187.9088347589046748, 138.8287307560422903, 1.515441477536284109 ) ) ;
#3117=CARTESIAN_POINT ( 'NONE',  ( -187.3343951027933656, 121.3449523462597313, -0.4555467707853332882 ) ) ;
#3128=CARTESIAN_POINT ( 'NONE',  ( -211.5791133502170283, 138.9897555992265268, 9.577123744044227394 ) ) ;
#3132=EDGE_CURVE ( 'NONE', #4070, #8499, #142, .T. ) ;
#3141=CARTESIAN_POINT ( 'NONE',  ( -172.7942878933874908, 118.6445810460862873, 8.630634598295349846 ) ) ;
#3142=CARTESIAN_POINT ( 'NONE',  ( -220.5827524467639762, 152.0305861332991526, -2.167411311894018144 ) ) ;
#3148=CARTESIAN_POINT ( 'NONE',  ( -222.6481022377596446, 148.3301877775025162, -2.885485496913823056 ) ) ;
#3188=CARTESIAN_POINT ( 'NONE',  ( -175.7692568323954845, 129.7291524912800185, -2.973479603620230893 ) ) ;
#3191=CARTESIAN_POINT ( 'NONE',  ( -175.8505196906716890, 123.8775902107358036, -5.297343846388533173 ) ) ;
#3202=CARTESIAN_POINT ( 'NONE',  ( -220.6842914767384229, 151.8486630221608209, 9.556866313350491637 ) ) ;
#3209=CARTESIAN_POINT ( 'NONE',  ( -222.5463326935617658, 144.4088500683630514, 2.431557144026069928 ) ) ;
#3213=CARTESIAN_POINT ( 'NONE',  ( -173.5807750188128296, 117.2354659032339299, 6.976364879781497663 ) ) ;
#3214=CARTESIAN_POINT ( 'NONE',  ( -222.6481022377693932, 148.3301877774849800, -2.885485496940157990 ) ) ;
#3223=CARTESIAN_POINT ( 'NONE',  ( -224.4522725256417743, 145.0977334997998014, 0.6248101478054410851 ) ) ;
#3235=EDGE_LOOP ( 'NONE', ( #1919, #2596 ) ) ;
#3244=DIRECTION ( 'NONE',  ( 0.8731965799097684000, -0.4873681696970819655, -0.000000000000000000 ) ) ;
#3249=CARTESIAN_POINT ( 'NONE',  ( -223.5985612785965486, 142.0411530078025635, 1.742203648027802254 ) ) ;
#3252=ORIENTED_EDGE ( 'NONE', *, *, #9048, .F. ) ;
#3265=CARTESIAN_POINT ( 'NONE',  ( -204.1471980322648960, 142.4963817258166614, -4.640918829492428621 ) ) ;
#3269=CARTESIAN_POINT ( 'NONE',  ( -194.2672495621651478, 127.5518908598051127, -0.4555467707853320669 ) ) ;
#3277=DIRECTION ( 'NONE',  ( 0.8731965799097682890, -0.4873681696970819099, 0.000000000000000000 ) ) ;
#3288=CARTESIAN_POINT ( 'NONE',  ( -210.0240857098682454, 141.7683007401625446, 10.16010209732750624 ) ) ;
#3301=CARTESIAN_POINT ( 'NONE',  ( -174.0007056342363683, 116.4830942877151756, 5.347843459918403930 ) ) ;
#3302=CARTESIAN_POINT ( 'NONE',  ( -224.7501301915791601, 144.5640747355008671, -2.630842070996033399 ) ) ;
#3328=CARTESIAN_POINT ( 'NONE',  ( -224.6003768274171080, 144.8323813947157817, 2.186315064719954737 ) ) ;
#3349=CARTESIAN_POINT ( 'NONE',  ( -192.4489746382803048, 130.7761537121523361, -4.642206099735005864 ) ) ;
#3365=CARTESIAN_POINT ( 'NONE',  ( -176.6594047394515314, 116.7136007993067324, 3.281269053145625225 ) ) ;
#3376=CARTESIAN_POINT ( 'NONE',  ( -223.7005213066090334, 146.4446138137323317, -1.719282361323794861 ) ) ;
#3394=CARTESIAN_POINT ( 'NONE',  ( -172.4561068142338058, 130.1936157287141498, 2.500000000515479215 ) ) ;
#3422=DIRECTION ( 'NONE',  ( 0.000000000000000000, 0.9953381730041138686, 0.09644646888731951695 ) ) ;
#3425=CARTESIAN_POINT ( 'NONE',  ( -212.8881127827856687, 136.6510672405775892, -2.964974570226852624 ) ) ;
#3433=B_SPLINE_CURVE_WITH_KNOTS ( 'NONE', 3,
 ( #15134, #15051, #5364, #4166, #6486, #4406, #5446, #766, #9235, #3079, #7908, #2998, #6719, #10183, #11522, #13964, #11283, #11442, #5525, #4095, #4325, #10260, #8928, #9165, #3148, #13885, #7981, #12768, #1725, #5604, #13722, #10416, #15211, #14033, #2925, #7748, #3223, #8060, #1649, #443 ),
 .UNSPECIFIED., .F., .F.,
 ( 4, 2, 2, 2, 2, 2, 2, 2, 2, 2, 2, 2, 2, 2, 2, 2, 2, 2, 2, 4 ),
 ( 0.01642013739010526191, 0.01748450029317128937, 0.01854886319623732030, 0.01961322609930334776, 0.02067758900236937869, 0.02120977045390238375, 0.02174195190543538880, 0.02280631480850148565, 0.02387067771156758250, 0.02493504061463367588, 0.02599940351769977273, 0.02653158496923285758, 0.02706376642076593897, 0.02812812932383207051, 0.02919249222689820206, 0.03025685512996433013, 0.03132121803303045821, 0.03185339948456353265, 0.03238558093609660016, 0.03344994383916276293 ),
 .UNSPECIFIED. ) ;
#3440=CARTESIAN_POINT ( 'NONE',  ( -199.4124801547868913, 127.6177204676982910, 1.515400478619089109 ) ) ;
#3454=CARTESIAN_POINT ( 'NONE',  ( -222.2186395530536629, 144.7337101510026116, -3.675081463328696341 ) ) ;
#3455=CARTESIAN_POINT ( 'NONE',  ( -219.3831369218127065, 150.1479396093025684, 9.707727764924111824 ) ) ;
#3462=SHAPE_REPRESENTATION_RELATIONSHIP ( 'NONE' , 'NONE' ,  #13652, #10185 ) ;
#3476=CARTESIAN_POINT ( 'NONE',  ( -223.5918188539070002, 142.0538562971642307, 1.612306317632525410 ) ) ;
#3499=CARTESIAN_POINT ( 'NONE',  ( -218.4400809351218413, 155.8695184890967482, 1.515441477806783510 ) ) ;
#3516=CARTESIAN_POINT ( 'NONE',  ( -181.9060177919747048, 118.7341819232202909, 5.367833425961690885 ) ) ;
#3529=CARTESIAN_POINT ( 'NONE',  ( -223.4760924884873248, 146.8467132707474434, -4.490349463211885883 ) ) ;
#3533=EDGE_CURVE ( 'NONE', #8499, #9526, #13673, .T. ) ;
#3534=CARTESIAN_POINT ( 'NONE',  ( -217.8113179378289317, 152.9593294075854431, 7.845513341075405656 ) ) ;
#3559=CARTESIAN_POINT ( 'NONE',  ( -223.3756880201893580, 142.5055725410610705, 5.363114072299179469 ) ) ;
#3564=CIRCLE ( 'NONE', #9622, 2.000000000000002220 ) ;
#3567=DIRECTION ( 'NONE',  ( -0.4873681696970817989, -0.8731965799097684000, 0.000000000000000000 ) ) ;
#3581=CARTESIAN_POINT ( 'NONE',  ( -206.2168697392640695, 148.5706983463157940, -0.4547266291960757045 ) ) ;
#3582=UNCERTAINTY_MEASURE_WITH_UNIT (LENGTH_MEASURE( 1.000000000000000082E-05 ), #13313, 'distance_accuracy_value', 'NONE');
#3597=CARTESIAN_POINT ( 'NONE',  ( -191.4964613557999655, 125.7493975051623352, 1.515400478619084224 ) ) ;
#3600=CARTESIAN_POINT ( 'NONE',  ( -209.3130641152695830, 145.0632059852189570, 9.578254705571840333 ) ) ;
#3627=CARTESIAN_POINT ( 'NONE',  ( -193.7200834347810599, 142.0619459586758921, 2.500000000000000000 ) ) ;
#3636=CARTESIAN_POINT ( 'NONE',  ( -223.1853449316457159, 142.8873074582503193, 6.221962389395381265 ) ) ;
#3651=CARTESIAN_POINT ( 'NONE',  ( -218.4444600228138711, 155.8616726660956715, 2.500000000270498735 ) ) ;
#3655=CARTESIAN_POINT ( 'NONE',  ( -206.0135413368010404, 148.9337379340180405, 1.515441477536285220 ) ) ;
#3670=CARTESIAN_POINT ( 'NONE',  ( -205.7735142771631160, 131.5899501701119334, 5.434137442415934771 ) ) ;
#3673=CARTESIAN_POINT ( 'NONE',  ( -179.6920193139674780, 128.7453118898713456, 9.578254705571842109 ) ) ;
#3697=CARTESIAN_POINT ( 'NONE',  ( -171.4541674549778918, 121.0456171749203662, 2.431557144026069928 ) ) ;
#3703=CARTESIAN_POINT ( 'NONE',  ( -201.8658614229783268, 146.6084512934502584, 2.500000000000000000 ) ) ;
#3710=CARTESIAN_POINT ( 'NONE',  ( -222.6541231320287579, 148.3194004002985196, 7.781232655114622254 ) ) ;
#3733=CARTESIAN_POINT ( 'NONE',  ( -207.9521514620915639, 147.4834172152791325, -2.963320117457100888 ) ) ;
#3751=CARTESIAN_POINT ( 'NONE',  ( -190.6388552492889517, 127.3288340616119143, -2.964974570226841522 ) ) ;
#3754=CARTESIAN_POINT ( 'NONE',  ( -211.5791133502170283, 138.9897555992265268, 9.577123744044227394 ) ) ;
#3765=CARTESIAN_POINT ( 'NONE',  ( -224.4522725255073397, 145.0977335000406470, 0.6248101478677640097 ) ) ;
#3782=ADVANCED_FACE ( 'NONE', ( #58 ), #2979, .T. ) ;
#3792=CARTESIAN_POINT ( 'NONE',  ( -219.9686238450918552, 153.1308939251236154, 5.827571112376363160 ) ) ;
#3794=CARTESIAN_POINT ( 'NONE',  ( -220.5676733911498388, 147.9555285791823849, 9.924366136672199801 ) ) ;
#3818=CARTESIAN_POINT ( 'NONE',  ( -186.0388298304660282, 135.7737150272329529, -2.963320117457103109 ) ) ;
#3835=CARTESIAN_POINT ( 'NONE',  ( -178.4226240946890130, 124.9752285324798606, -5.265047855996060733 ) ) ;
#3837=CARTESIAN_POINT ( 'NONE',  ( -204.9546745879972889, 133.0893851581147374, 7.918248976830629893 ) ) ;
#3853=CARTESIAN_POINT ( 'NONE',  ( -188.8176989649505231, 137.2180184133358694, 7.919662025281898998 ) ) ;
#3864=CARTESIAN_POINT ( 'NONE',  ( -207.9892458934089632, 147.4169567187306029, 7.919662025281897222 ) ) ;
#3869=CARTESIAN_POINT ( 'NONE',  ( -222.2279178565764255, 149.0830140542140043, 7.930883854505606401 ) ) ;
#3872=CARTESIAN_POINT ( 'NONE',  ( -220.1006191622630297, 148.8276055330639736, 9.939501965825337848 ) ) ;
#3874=CARTESIAN_POINT ( 'NONE',  ( -173.8777679508388019, 116.7033564454829673, -1.424210617517640554 ) ) ;
#3905=CARTESIAN_POINT ( 'NONE',  ( -222.7490783815899533, 143.6991938219488247, -2.614991558308088937 ) ) ;
#3906=CARTESIAN_POINT ( 'NONE',  ( -214.7080733591933779, 145.5905563435376848, -5.230826428279589990 ) ) ;
#3909=CARTESIAN_POINT ( 'NONE',  ( -168.3973611425364822, 125.8284172634911755, 7.880738923213935543 ) ) ;
#3922=CARTESIAN_POINT ( 'NONE',  ( -167.6801169734147265, 127.1165587117766336, 5.426559898713293251 ) ) ;
#3936=CARTESIAN_POINT ( 'NONE',  ( -211.4864660300886499, 151.5260579444296525, 5.434754235172608361 ) ) ;
#3943=CARTESIAN_POINT ( 'NONE',  ( -222.4836136237429116, 148.6248949498702530, 7.868731570916820850 ) ) ;
#3945=CARTESIAN_POINT ( 'NONE',  ( -220.2521499497359230, 152.6229124025628323, 6.494025194934711642 ) ) ;
#3972=CARTESIAN_POINT ( 'NONE',  ( -219.1618877908461513, 150.5179266800831215, -4.694150837216314542 ) ) ;
#3974=CARTESIAN_POINT ( 'NONE',  ( -197.2022238459480263, 131.7665462075744358, -4.642206099735013858 ) ) ;
#3977=CARTESIAN_POINT ( 'NONE',  ( -205.7735142771631160, 131.5899501701119334, 5.434137442415934771 ) ) ;
#3989=CARTESIAN_POINT ( 'NONE',  ( -193.7244371550166022, 142.0541455854551600, 3.478855109513427468 ) ) ;
#4005=CARTESIAN_POINT ( 'NONE',  ( -219.4404776672114963, 154.0771507077609499, 1.641297965848094842 ) ) ;
#4006=CARTESIAN_POINT ( 'NONE',  ( -170.1156333370428229, 128.4548013739684791, 5.428578397873499384 ) ) ;
#4017=CARTESIAN_POINT ( 'NONE',  ( -222.1940576498694213, 149.1436799296412801, 9.935665413336629115 ) ) ;
#4019=CARTESIAN_POINT ( 'NONE',  ( -168.5042799224661110, 126.3308037436463849, -2.295422687810467099 ) ) ;
#4040=CARTESIAN_POINT ( 'NONE',  ( -187.9132138465967898, 138.8208849330412988, 2.500000000000000000 ) ) ;
#4055=CARTESIAN_POINT ( 'NONE',  ( -216.7768923448186342, 154.7526869307816071, 0.8713118593939417345 ) ) ;
#4056=CARTESIAN_POINT ( 'NONE',  ( -220.6443225159919734, 151.9202736894074803, -4.662307221713795968 ) ) ;
#4058=VERTEX_POINT ( 'NONE', #8006 ) ;
#4059=CARTESIAN_POINT ( 'NONE',  ( -176.4886329031608909, 117.0201139606268441, 5.242686462712208062 ) ) ;
#4070=VERTEX_POINT ( 'NONE', #13100 ) ;
#4073=CARTESIAN_POINT ( 'NONE',  ( -170.1156333370428229, 128.4548013739684791, 5.428578397873499384 ) ) ;
#4089=CARTESIAN_POINT ( 'NONE',  ( -218.3154676233766338, 152.0521266355204091, -3.827015397074207570 ) ) ;
#4095=CARTESIAN_POINT ( 'NONE',  ( -221.8782673190674188, 149.7094678780368042, -3.059957786096294097 ) ) ;
#4097=CARTESIAN_POINT ( 'NONE',  ( -218.8494421554486848, 151.1141414623175763, 9.296710778528519015 ) ) ;
#4131=CARTESIAN_POINT ( 'NONE',  ( -172.5271923976867470, 129.8359673051191123, -0.4588839673349612291 ) ) ;
#4134=CARTESIAN_POINT ( 'NONE',  ( -199.4124801547868913, 127.6177204676982910, 3.478895870929493483 ) ) ;
#4146=CARTESIAN_POINT ( 'NONE',  ( -194.7616377892423714, 140.1172406977107130, 7.919662025281898998 ) ) ;
#4157=CARTESIAN_POINT ( 'NONE',  ( -220.3531759299249302, 148.3382346779569616, 2.431557144026069928 ) ) ;
#4158=CARTESIAN_POINT ( 'NONE',  ( -218.4677351830677878, 155.8199715629169475, 3.280001329127711251 ) ) ;
#4166=CARTESIAN_POINT ( 'NONE',  ( -219.4404776675327184, 154.0771507071854671, 1.641297965941626247 ) ) ;
#4168=CARTESIAN_POINT ( 'NONE',  ( -219.1310489671168114, 154.6315407961138249, 6.827724881366695975 ) ) ;
#4170=CARTESIAN_POINT ( 'NONE',  ( -172.4948715304248594, 119.1810324607742615, -4.416274670461012519 ) ) ;
#4205=CARTESIAN_POINT ( 'NONE',  ( -186.0388298304660282, 135.7737150272329529, -2.963320117457103109 ) ) ;
#4208=CARTESIAN_POINT ( 'NONE',  ( -173.7799404587539698, 116.1630799793301350, 5.180112981087466650 ) ) ;
#4221=CARTESIAN_POINT ( 'NONE',  ( -189.6066827460468858, 129.2255495722319836, 9.577123744044220288 ) ) ;
#4234=CARTESIAN_POINT ( 'NONE',  ( -168.6364115625881084, 126.0940691691992441, 7.458761130116111637 ) ) ;
#4283=EDGE_CURVE ( 'NONE', #9509, #4058, #146, .T. ) ;
#4284=CARTESIAN_POINT ( 'NONE',  ( -195.9617019660094570, 137.8802668252396586, -4.640918829492428621 ) ) ;
#4288=CARTESIAN_POINT ( 'NONE',  ( -198.8906912147545540, 132.4339616203728838, -4.642206099735012970 ) ) ;
#4303=CARTESIAN_POINT ( 'NONE',  ( -175.8847466161772957, 123.8162673009714752, 10.09358467921856573 ) ) ;
#4316=CARTESIAN_POINT ( 'NONE',  ( -220.4428784760110034, 152.2811923084124714, -1.958540667413632974 ) ) ;
#4325=CARTESIAN_POINT ( 'NONE',  ( -222.0498794291112290, 149.4019978443362220, -3.065875947101888599 ) ) ;
#4365=CARTESIAN_POINT ( 'NONE',  ( -179.9223906590855222, 134.3711564447467310, 1.515441477536284554 ) ) ;
#4368=CARTESIAN_POINT ( 'NONE',  ( -197.2022238459480263, 131.7665462075744358, -4.642206099735013858 ) ) ;
#4374=DIRECTION ( 'NONE',  ( 0.4873681696970831312, 0.8731965799097676229, 0.000000000000000000 ) ) ;
#4384=CARTESIAN_POINT ( 'NONE',  ( -217.2220691230952525, 140.9637235289241062, 7.918248976830628116 ) ) ;
#4396=CARTESIAN_POINT ( 'NONE',  ( -221.3196620123036951, 146.4694855639384912, -4.679075448335836107 ) ) ;
#4406=CARTESIAN_POINT ( 'NONE',  ( -219.5587625783448971, 153.8652247218668379, 0.6104961446958759863 ) ) ;
#4441=CARTESIAN_POINT ( 'NONE',  ( -218.6225377568032684, 155.5426184521650441, -0.4568654681747655322 ) ) ;
#4445=CARTESIAN_POINT ( 'NONE',  ( -176.4863952559862526, 117.0241230567913959, -0.6469977504890583875 ) ) ;
#4458=CARTESIAN_POINT ( 'NONE',  ( -208.4664676862339832, 144.5514869593766036, 9.578254705571838556 ) ) ;
#4469=CARTESIAN_POINT ( 'NONE',  ( -167.8263066260882397, 127.5454993279624745, 3.430700028191667084 ) ) ;
#4470=CARTESIAN_POINT ( 'NONE',  ( -224.9839264852863323, 144.1451919755143081, -2.062628029334759638 ) ) ;
#4516=B_SPLINE_CURVE_WITH_KNOTS ( 'NONE', 3,
 ( #14243, #13048, #7085, #1686, #11177, #328, #12344, #9758, #9916, #3905, #13599, #8805, #6282, #9997, #13448, #5168, #483, #2569, #6522, #13681, #1530, #11249, #14780, #2648, #7710, #3972, #7469, #12264, #12189, #405, #5017, #2808, #1442, #13522, #9840, #7629, #14636, #12421, #2723, #8728, #4055, #1369, #2886, #1612 ),
 .UNSPECIFIED., .F., .F.,
 ( 4, 2, 2, 2, 2, 2, 2, 2, 2, 2, 2, 2, 2, 2, 2, 2, 2, 2, 2, 2, 2, 4 ),
 ( 0.0008097935439387997673, 0.002225919271470510382, 0.002933982135236355010, 0.003642044999002200072, 0.005058170726533871113, 0.006474296454065542154, 0.007890422181597214063, 0.008598485045363033971, 0.009306547909128853879, 0.01072267363666049370, 0.01213879936419213178, 0.01284686222795791352, 0.01355492509172369700, 0.01497105081925522753, 0.01638717654678675806, 0.01780330227431829032, 0.01851136513808408421, 0.01921942800184987116, 0.02063555372938145199, 0.02134361659314724241, 0.02205167945691303283, 0.02346780518444461713 ),
 .UNSPECIFIED. ) ;
#4521=CARTESIAN_POINT ( 'NONE',  ( -172.3582205330567945, 130.1389812296867774, 2.500000000525777644 ) ) ;
#4525=CARTESIAN_POINT ( 'NONE',  ( -177.2366359034146512, 121.3924996022181375, -4.733667549831950261 ) ) ;
#4544=CARTESIAN_POINT ( 'NONE',  ( -172.0064303153328638, 119.3480080297071595, 9.396848320176498959 ) ) ;
#4557=CARTESIAN_POINT ( 'NONE',  ( -221.6351743891050603, 145.8627096086362371, -4.407674936793750220 ) ) ;
#4558=CARTESIAN_POINT ( 'NONE',  ( -221.3451643498282806, 146.4827145868442528, 9.580214341060731442 ) ) ;
#4568=CARTESIAN_POINT ( 'NONE',  ( 0.000000000000000000, 0.000000000000000000, 0.000000000000000000 ) ) ;
#4573=CARTESIAN_POINT ( 'NONE',  ( -177.3557003870508595, 132.9282874014947140, 2.500000000000000000 ) ) ;
#4606=CARTESIAN_POINT ( 'NONE',  ( -209.9898587843626956, 141.8296236499265035, -5.230826428279598872 ) ) ;
#4621=CARTESIAN_POINT ( 'NONE',  ( -186.4931015233695462, 122.8215886266871593, 7.918248976830652097 ) ) ;
#4622=CARTESIAN_POINT ( 'NONE',  ( -219.4360840196855804, 154.0850226169901305, 3.058976617611859794 ) ) ;
#4632=CARTESIAN_POINT ( 'NONE',  ( -223.1312025536231261, 147.4646377276753242, -2.512173040697494475 ) ) ;
#4679=CARTESIAN_POINT ( 'NONE',  ( -170.8299300849453459, 127.1729693371208043, -2.992655347556774981 ) ) ;
#4696=CARTESIAN_POINT ( 'NONE',  ( -173.7799404587539698, 116.1630799793301350, 5.180112981087466650 ) ) ;
#4706=CARTESIAN_POINT ( 'NONE',  ( -213.9960106562366491, 134.6720553025416507, 2.431555724346858849 ) ) ;
#4710=CARTESIAN_POINT ( 'NONE',  ( -223.2496967378148724, 147.2523367962785414, -4.668145987003846642 ) ) ;
#4737=CARTESIAN_POINT ( 'NONE',  ( -225.5877652983326982, 143.0633199552225960, 4.273891064090742375 ) ) ;
#4745=( GEOMETRIC_REPRESENTATION_CONTEXT ( 3 ) GLOBAL_UNCERTAINTY_ASSIGNED_CONTEXT ( ( #3582 ) ) GLOBAL_UNIT_ASSIGNED_CONTEXT ( ( #13313, #6153, #10654 ) ) REPRESENTATION_CONTEXT ( 'NONE', 'WORKASPACE' ) );
#4761=CARTESIAN_POINT ( 'NONE',  ( -167.6561596704311512, 127.1594819807359329, -0.4629209656553701646 ) ) ;
#4778=CARTESIAN_POINT ( 'NONE',  ( -221.7331157600676192, 141.5908957077777188, 3.478895870929496148 ) ) ;
#4782=CARTESIAN_POINT ( 'NONE',  ( -179.8866491758529094, 122.3521977864031243, 9.530069280832647038 ) ) ;
#4783=CARTESIAN_POINT ( 'NONE',  ( -167.7990583880505824, 127.5943188236592363, 2.500000001005440620 ) ) ;
#4814=CARTESIAN_POINT ( 'NONE',  ( -201.8702151432138692, 146.6006509202294410, 3.478855109513426580 ) ) ;
#4823=CARTESIAN_POINT ( 'NONE',  ( -222.9850097917987171, 147.7265650088764346, 7.563253245014972315 ) ) ;
#4825=ORIENTED_EDGE ( 'NONE', *, *, #1378, .T. ) ;
#4838=ORIENTED_EDGE ( 'NONE', *, *, #5398, .T. ) ;
#4848=CARTESIAN_POINT ( 'NONE',  ( -192.3464331062453709, 140.8629472311621100, -0.4547266291960749829 ) ) ;
#4863=CARTESIAN_POINT ( 'NONE',  ( -184.9748306402843809, 119.2867206268225999, 1.515400478619091995 ) ) ;
#4867=CARTESIAN_POINT ( 'NONE',  ( -204.1871669930114024, 142.4247710585700020, 9.578254705571842109 ) ) ;
#4872=CARTESIAN_POINT ( 'NONE',  ( -191.4963330474078020, 125.7496346496455004, 2.431555724346856184 ) ) ;
#4878=CARTESIAN_POINT ( 'NONE',  ( -217.4370776556141607, 153.6126725021986772, 6.955470517783211903 ) ) ;
#4883=CARTESIAN_POINT ( 'NONE',  ( -211.2987210398670186, 151.8733316563206586, 2.500000000000000000 ) ) ;
#4897=CARTESIAN_POINT ( 'NONE',  ( -211.3030747601025610, 151.8655312830997559, 3.478855109513426580 ) ) ;
#4907=CARTESIAN_POINT ( 'NONE',  ( -222.0618215705420369, 145.1005326155232922, 8.841470136485687803 ) ) ;
#4916=FACE_OUTER_BOUND ( 'NONE', #1053, .T. ) ;
#4927=CARTESIAN_POINT ( 'NONE',  ( -188.0666105031049824, 138.5497687542270739, -0.4547266291960739282 ) ) ;
#4939=CARTESIAN_POINT ( 'NONE',  ( -181.0860728093183809, 120.2032420692993071, -3.023257939496618807 ) ) ;
#4943=CARTESIAN_POINT ( 'NONE',  ( -197.2254974982137128, 131.7248478061943615, 9.577123744044225617 ) ) ;
#4959=CARTESIAN_POINT ( 'NONE',  ( -179.9267697467775520, 134.3633106217456543, 2.500000000000000000 ) ) ;
#4970=CARTESIAN_POINT ( 'NONE',  ( -185.2098801967860595, 137.3018090142982146, 3.478855109513427468 ) ) ;
#4979=CARTESIAN_POINT ( 'NONE',  ( -222.4011748855326687, 148.7725968900727764, 7.888572101362996136 ) ) ;
#4981=ADVANCED_FACE ( 'NONE', ( #15311 ), #15471, .T. ) ;
#5001=CARTESIAN_POINT ( 'NONE',  ( -177.3513212993587729, 132.9361332244957055, 1.515441477536284109 ) ) ;
#5002=CARTESIAN_POINT ( 'NONE',  ( -223.6090965991043902, 142.0216235376909424, 2.002380365345714619 ) ) ;
#5010=EDGE_LOOP ( 'NONE', ( #11215, #5717 ) ) ;
#5017=CARTESIAN_POINT ( 'NONE',  ( -217.8165228275882157, 152.9407092898246958, -2.993413372942824502 ) ) ;
#5018=CARTESIAN_POINT ( 'NONE',  ( -178.4115273750087738, 119.2860570028907858, -3.078262048313290311 ) ) ;
#5021=CARTESIAN_POINT ( 'NONE',  ( -194.3889542450793613, 137.0335258394182745, 9.578254705571838556 ) ) ;
#5034=CARTESIAN_POINT ( 'NONE',  ( -211.4864660300886499, 151.5260579444296525, 5.434754235172608361 ) ) ;
#5047=CARTESIAN_POINT ( 'NONE',  ( -174.7846310273254176, 131.4932641812416421, 2.500000000270498735 ) ) ;
#5055=CARTESIAN_POINT ( 'NONE',  ( -224.4579709560119909, 145.0875238672886951, 4.289685626893874115 ) ) ;
#5057=CARTESIAN_POINT ( 'NONE',  ( -221.7730551926511566, 145.6605518061857083, 9.210365250596908027 ) ) ;
#5059=CARTESIAN_POINT ( 'NONE',  ( -173.2963660003902362, 117.7450293044227294, -3.133322902959446932 ) ) ;
#5094=CARTESIAN_POINT ( 'NONE',  ( -189.5834090937817109, 129.2672479736120010, -4.642206099735012970 ) ) ;
#5097=CARTESIAN_POINT ( 'NONE',  ( -220.6842914767384229, 151.8486630221608209, 9.556866313350491637 ) ) ;
#5105=CARTESIAN_POINT ( 'NONE',  ( -224.3206423881711089, 145.3335695535245975, -0.03206942349657965208 ) ) ;
#5110=CARTESIAN_POINT ( 'NONE',  ( -178.4232521731099439, 131.0169814278324907, 7.919662025281895446 ) ) ;
#5126=CARTESIAN_POINT ( 'NONE',  ( -215.8266853215729668, 152.1588074852305112, 7.919662025281898998 ) ) ;
#5134=CARTESIAN_POINT ( 'NONE',  ( -218.4292495602899749, 151.8671251436307159, 8.843529103934264057 ) ) ;
#5136=CARTESIAN_POINT ( 'NONE',  ( -167.7990583880505824, 127.5943188236592363, 2.500000001005440620 ) ) ;
#5144=ORIENTED_EDGE ( 'NONE', *, *, #765, .T. ) ;
#5156=CARTESIAN_POINT ( 'NONE',  ( -193.7200834347810599, 142.0619459586758921, 2.500000000000000000 ) ) ;
#5168=CARTESIAN_POINT ( 'NONE',  ( -221.5309300683038032, 146.0635204735091293, -4.506196516310935429 ) ) ;
#5169=CARTESIAN_POINT ( 'NONE',  ( -220.7908126485560274, 143.2766720833714089, -2.964974570226855288 ) ) ;
#5174=CARTESIAN_POINT ( 'NONE',  ( -173.9416064256852508, 115.8726071073731987, 1.253181679794994174 ) ) ;
#5188=CARTESIAN_POINT ( 'NONE',  ( -206.0222741447286126, 148.9180917377961464, 3.478855109513426580 ) ) ;
#5200=CARTESIAN_POINT ( 'NONE',  ( -218.4373823716798597, 155.8743533890948356, 2.316433880752911012 ) ) ;
#5201=CARTESIAN_POINT ( 'NONE',  ( -202.0760438715631437, 146.2294067514662288, 5.434754235172608361 ) ) ;
#5208=CARTESIAN_POINT ( 'NONE',  ( -219.7781685404717393, 153.4721244997903398, 5.234562638556204739 ) ) ;
#5210=CARTESIAN_POINT ( 'NONE',  ( -220.6620190085783406, 151.8885676450574636, 7.148697176988450863 ) ) ;
#5212=CARTESIAN_POINT ( 'NONE',  ( -169.2883314711424134, 124.9260523188610392, -3.943474352876168876 ) ) ;
#5233=CARTESIAN_POINT ( 'NONE',  ( -205.9650630239422640, 131.2381394179032839, 2.431555724346861957 ) ) ;
#5243=CARTESIAN_POINT ( 'NONE',  ( -198.4137021260360711, 129.4968702780754199, -2.964974570226842410 ) ) ;
#5246=CARTESIAN_POINT ( 'NONE',  ( -184.9748306402843809, 119.2867206268225999, 1.515400478619091995 ) ) ;
#5252=DIRECTION ( 'NONE',  ( 0.8731965799097682890, -0.4873681696970819099, 0.000000000000000000 ) ) ;
#5255=B_SPLINE_CURVE_WITH_KNOTS ( 'NONE', 3,
 ( #1793, #6710, #14099, #13877, #6863, #11514, #3301, #756, #13953, #8136, #3213, #6780, #1942, #12921, #5596, #3141, #10406, #15275, #2989, #2108, #6942, #15351, #8051, #9072, #5514, #10250, #10485, #11674, #7971, #671, #11590, #3069, #12759, #599, #12681, #10330, #15201, #4234, #15043, #835, #15124, #10558, #9227, #12837, #7897, #5670, #4469, #1868, #5743, #11749 ),
 .UNSPECIFIED., .F., .F.,
 ( 4, 2, 2, 2, 2, 2, 2, 2, 2, 2, 2, 2, 2, 2, 2, 2, 2, 2, 2, 2, 2, 2, 2, 2, 4 ),
 ( 0.04400301569768626936, 0.04538375231244021896, 0.04676448892719416855, 0.04745485723457115029, 0.04814522554194812509, 0.04952596215670206081, 0.05021633046407901479, 0.05090669877145596878, 0.05228743538620987674, 0.05297780369358683072, 0.05366817200096378471, 0.05435854030834073175, 0.05504890861571768573, 0.05642964523047158676, 0.05712001353784854768, 0.05781038184522550166, 0.05850075015260245564, 0.05919111845997940963, 0.06057185507473332453, 0.06126222338211030627, 0.06195259168948728801, 0.06333332830424129312, 0.06471406491899528435, 0.06540443322637229384, 0.06609480153374930333 ),
 .UNSPECIFIED. ) ;
#5259=CARTESIAN_POINT ( 'NONE',  ( -202.0760438715631437, 146.2294067514662288, 5.434754235172608361 ) ) ;
#5272=CARTESIAN_POINT ( 'NONE',  ( -219.5883309621183628, 153.8122483208824463, -3.038090696635943999 ) ) ;
#5287=CARTESIAN_POINT ( 'NONE',  ( -220.9667893534755194, 151.3425237312999911, 7.477333657888038942 ) ) ;
#5307=CARTESIAN_POINT ( 'NONE',  ( -172.3538414453648500, 130.1468270526879110, 1.515441478062062641 ) ) ;
#5323=CARTESIAN_POINT ( 'NONE',  ( -209.2730951545231335, 145.1348166524657302, -4.640918829492436615 ) ) ;
#5327=CARTESIAN_POINT ( 'NONE',  ( -182.0950013669840359, 118.3955881831737997, 3.410453015226076801 ) ) ;
#5341=CARTESIAN_POINT ( 'NONE',  ( -187.9175675668324175, 138.8130845598205667, 3.478855109513427468 ) ) ;
#5356=CARTESIAN_POINT ( 'NONE',  ( -216.7684744367785186, 154.7672370854363635, 0.8965377175049941139 ) ) ;
#5364=CARTESIAN_POINT ( 'NONE',  ( -219.4139989651374947, 154.1245914589817119, 2.346545548906505907 ) ) ;
#5366=CARTESIAN_POINT ( 'NONE',  ( -216.7978016317474044, 154.7161345818039422, 4.230144757024230984 ) ) ;
#5371=CARTESIAN_POINT ( 'NONE',  ( -168.3799913776774133, 126.5534861816458800, -1.907514191769585921 ) ) ;
#5392=CARTESIAN_POINT ( 'NONE',  ( -172.3582205330567945, 130.1389812296867774, 2.500000000525777644 ) ) ;
#5393=CARTESIAN_POINT ( 'NONE',  ( -217.6896908598658911, 153.1102862775958897, 3.058976617611858906 ) ) ;
#5398=EDGE_CURVE ( 'NONE', #13381, #9509, #6124, .T. ) ;
#5408=CARTESIAN_POINT ( 'NONE',  ( -171.9495551447802200, 125.1641050887067053, -4.702677209512893697 ) ) ;
#5411=CARTESIAN_POINT ( 'NONE',  ( -178.4228374502453107, 119.2657932277225967, 7.804961498744191317 ) ) ;
#5424=CARTESIAN_POINT ( 'NONE',  ( -168.3973611425364822, 125.8284172634911755, 7.880738923213935543 ) ) ;
#5436=CARTESIAN_POINT ( 'NONE',  ( -220.2506544536004469, 152.6255918186425617, -1.607790317125668222 ) ) ;
#5446=CARTESIAN_POINT ( 'NONE',  ( -219.6200563868712266, 153.7554072423868661, 0.2735799752493159875 ) ) ;
#5448=CARTESIAN_POINT ( 'NONE',  ( -219.2006734968679211, 154.5067975218504444, 7.020207066939610385 ) ) ;
#5487=CARTESIAN_POINT ( 'NONE',  ( -207.0700983879231387, 149.0508413170868209, -0.4547266291960758156 ) ) ;
#5490=CARTESIAN_POINT ( 'NONE',  ( -225.7548303624725179, 142.7639966680278576, 3.410453015226076801 ) ) ;
#5500=CARTESIAN_POINT ( 'NONE',  ( -177.0244624812495999, 127.4802545373068767, 9.556866313350486308 ) ) ;
#5503=B_SPLINE_SURFACE_WITH_KNOTS ( 'NONE', 3, 3, ( 
 ( #5986, #13230, #4883, #2430, #1000, #9702, #1316, #13074, #11989, #13152, #14567, #4959, #9774, #7025, #11832, #10649, #9466 ),
 ( #1549, #14727, #6384, #11192, #5188, #13467, #500, #3989, #2904, #5341, #7727, #14796, #11268, #13536, #8823, #1385, #10085 ),
 ( #271, #6299, #5034, #13701, #2667, #5259, #11116, #13618, #7485, #2825, #12279, #7647, #12439, #14878, #12514, #4073, #3922 ),
 ( #6540, #6223, #10163, #14955, #9860, #8745, #9936, #4146, #14652, #3853, #1460, #8674, #5110, #2742, #7565, #15262, #5424 ),
 ( #3202, #824, #11575, #9143, #4458, #9290, #12747, #8037, #10545, #11504, #14087, #15032, #15111, #5500, #742, #11663, #6931 ),
 ( #6851, #1856, #10317, #7886, #3288, #7805, #5733, #12909, #10395, #661, #6621, #11420, #12825, #5658, #4303, #8122, #1932 ),
 ( #13941, #13779, #2013, #2098, #3128, #6699, #12668, #7959, #10475, #11738, #4221, #901, #586, #5584, #9059, #13865, #4544 ),
 ( #15340, #15189, #4384, #2976, #12592, #6768, #1782, #9215, #10240, #3057, #14012, #4621, #15499, #12039, #5889, #2251, #12116 ),
 ( #7168, #10707, #10948, #9449, #8433, #10871, #3670, #1295, #10786, #15573, #11971, #9371, #9519, #3516, #13212, #2410, #4696 ),
 ( #13049, #4778, #99, #2173, #5809, #13288, #8204, #13134, #14317, #14399, #1212, #8353, #14244, #2336, #14167, #3365, #6128 ),
 ( #1140, #10629, #15421, #5967, #1066, #7086, #12983, #6050, #3440, #9603, #3597, #7245, #4863, #7320, #7003, #8273, #11891 ),
 ( #25, #11813, #9682, #978, #14475, #8504, #2488, #11178, #8892, #6445, #12190, #13682, #9998, #7630, #2725, #254, #11250 ),
 ( #9759, #5169, #7549, #2888, #7711, #8654, #12346, #14549, #5243, #14781, #3751, #13450, #1370, #4939, #5018, #2570, #13601 ),
 ( #12497, #14861, #14708, #1531, #2809, #330, #8579, #6367, #3974, #6208, #5094, #14637, #1687, #9843, #11019, #7470, #13523 ),
 ( #13372, #9918, #3906, #8806, #12422, #1444, #1614, #2649, #406, #11324, #7400, #170, #6524, #3835, #8729, #6283, #10068 ),
 ( #4056, #12265, #11099, #5323, #6909, #3265, #8106, #4284, #1767, #6603, #647, #7870, #9042, #485, #8018, #5408, #722 ),
 ( #6684, #11643, #14072, #12890, #10224, #570, #2076, #11487, #14941, #15018, #4205, #11559, #9124, #3188, #11404, #805, #12728 ),
 ( #4441, #10377, #15245, #5487, #15092, #12806, #13997, #9275, #10148, #9201, #13842, #12653, #3040, #5639, #4131, #8970, #13763 ),
 ( #1840, #2961, #7786, #15170, #1995, #10301, #10458, #13925, #12570, #3114, #7944, #4365, #6832, #1917, #6752, #5565, #2231 ),
 ( #3651, #13116, #2315, #14297, #11720, #11875, #5872, #15552, #10766, #8256, #11951, #15403, #7145, #2465, #4521, #8182, #6 ) ),
 .UNSPECIFIED., .T., .F., .F.,
 ( 4, 1, 1, 1, 1, 1, 1, 1, 2, 1, 1, 1, 1, 1, 1, 1, 4 ),
 ( 4, 2, 2, 2, 2, 2, 3, 4 ),
 ( 0.000000000000000000, 0.06231844716590150685, 0.1246368943318030137, 0.1869553414977045136, 0.2492737886636060274, 0.3115922358295075134, 0.3739106829954090272, 0.4362291301613105410, 0.4985475773272120548, 0.5612291301613105965, 0.6239106829954090827, 0.6865922358295075689, 0.7492737886636060551, 0.8119553414977045414, 0.8746368943318030276, 0.9373184471659015138, 1.000000000000000000 ),
 ( 0.000000000000000000, 0.2455027589669699362, 0.3041813370740077405, 0.5308033955276700855, 0.6372805264318514018, 0.8233339832829627003, 1.000000000000000000, 1.166726064904226812 ),
 .UNSPECIFIED. ) ;
#5512=( BOUNDED_SURFACE ( )  B_SPLINE_SURFACE ( 3, 2, ( 
 ( #2918, #4158, #6554 ),
 ( #3070, #358, #517 ),
 ( #6475, #5200, #15125 ),
 ( #7898, #12525, #4005 ),
 ( #5356, #2990, #10025 ),
 ( #10176, #13633, #11355 ),
 ( #6637, #13791, #10331 ),
 ( #10100, #7819, #11206 ),
 ( #7741, #600, #12682 ),
 ( #11278, #14966, #2838 ),
 ( #9156, #13954, #12608 ),
 ( #1794, #1716, #14893 ),
 ( #1869, #5272, #5436 ),
 ( #10251, #6711, #4316 ),
 ( #4089, #8920, #3142 ),
 ( #7659, #15044, #11515 ),
 ( #672, #5515, #12454 ),
 ( #7972, #6399, #5900 ),
 ( #1078, #12922, #914 ),
 ( #15433, #10719, #6782 ),
 ( #5671, #9305, #11675 ),
 ( #14101, #15352, #2109 ),
 ( #14258, #11591, #11750 ),
 ( #12840, #757, #15512 ),
 ( #8137, #1943, #992 ),
 ( #6943, #10486, #836 ),
 ( #9461, #5822, #3214 ),
 ( #4396, #9383, #8052 ),
 ( #8366, #4710, #11903 ),
 ( #4557, #3529, #5597 ),
 ( #11826, #5744, #4632 ),
 ( #9532, #14330, #10559 ),
 ( #3454, #12994, #10407 ),
 ( #14178, #9228, #3376 ),
 ( #15202, #6864, #14025 ),
 ( #8216, #2029, #15276 ),
 ( #2186, #3302, #7014 ),
 ( #10641, #4470, #8285 ),
 ( #13064, #2266, #7098 ),
 ( #14648, #7481, #5105 ),
 ( #14561, #112, #13146 ),
 ( #9697, #12132, #6141 ),
 ( #8444, #6293, #3765 ),
 ( #2501, #8516, #9931 ),
 ( #13302, #1308, #2348 ),
 ( #8592, #10884, #1228 ) ),
 .UNSPECIFIED., .F., .F., .T. ) 
 B_SPLINE_SURFACE_WITH_KNOTS ( ( 4, 2, 2, 2, 2, 2, 2, 2, 2, 2, 2, 2, 2, 2, 2, 2, 2, 2, 2, 2, 2, 2, 4 ),
 ( 3, 3 ),
 ( 0.01690353391188639809, 0.01796000478138011502, 0.01901647565087383543, 0.02007294652036755583, 0.02112941738986127277, 0.02165765282460813124, 0.02218588825935499317, 0.02324235912884871358, 0.02429882999834243051, 0.02482706543308928898, 0.02535530086783615092, 0.02641177173732987132, 0.02694000717207672979, 0.02746824260682358826, 0.02799647804157044673, 0.02852471347631730866, 0.02958118434581102907, 0.03010941978055788754, 0.03063765521530474600, 0.03169412608479846294, 0.03222236151954532141, 0.03275059695429217987, 0.03380706782378590375 ),
 ( 0.000000000000000000, 1.000000000000000000 ),
 .UNSPECIFIED. ) 
 GEOMETRIC_REPRESENTATION_ITEM ( )  RATIONAL_B_SPLINE_SURFACE ( (
 ( 1.000000000000000000, 0.7072571230116134755, 1.000000000000000000),
 ( 1.000000000000000000, 0.7070704586539242609, 1.000000000000000000),
 ( 1.000000000000000000, 0.7070624175750332974, 1.000000000000000000),
 ( 1.000000000000000000, 0.7073610487233381594, 1.000000000000000000),
 ( 1.000000000000000000, 0.7076621214645069102, 1.000000000000000000),
 ( 1.000000000000000000, 0.7084745963449632367, 1.000000000000000000),
 ( 1.000000000000000000, 0.7089917081225262097, 1.000000000000000000),
 ( 1.000000000000000000, 0.7100509560662205955, 1.000000000000000000),
 ( 1.000000000000000000, 0.7105995507477381734, 1.000000000000000000),
 ( 1.000000000000000000, 0.7113270099474451325, 1.000000000000000000),
 ( 1.000000000000000000, 0.7115528126308224843, 1.000000000000000000),
 ( 1.000000000000000000, 0.7119351551072216067, 1.000000000000000000),
 ( 1.000000000000000000, 0.7120930000513538971, 1.000000000000000000),
 ( 1.000000000000000000, 0.7124440185857547903, 1.000000000000000000),
 ( 1.000000000000000000, 0.7125154292520059496, 1.000000000000000000),
 ( 1.000000000000000000, 0.7121332859195406151, 1.000000000000000000),
 ( 1.000000000000000000, 0.7116646334020431119, 1.000000000000000000),
 ( 1.000000000000000000, 0.7105288043779220963, 1.000000000000000000),
 ( 1.000000000000000000, 0.7100784943464703014, 1.000000000000000000),
 ( 1.000000000000000000, 0.7090174157212792982, 1.000000000000000000),
 ( 1.000000000000000000, 0.7084074433244883506, 1.000000000000000000),
 ( 1.000000000000000000, 0.7063588986342012044, 1.000000000000000000),
 ( 1.000000000000000000, 0.7046589198606203475, 1.000000000000000000),
 ( 1.000000000000000000, 0.7017665165854515275, 1.000000000000000000),
 ( 1.000000000000000000, 0.7007370448553386089, 1.000000000000000000),
 ( 1.000000000000000000, 0.6986007619009740877, 1.000000000000000000),
 ( 1.000000000000000000, 0.6974911578170575055, 1.000000000000000000),
 ( 1.000000000000000000, 0.6951922021189940182, 1.000000000000000000),
 ( 1.000000000000000000, 0.6940027630648812895, 1.000000000000000000),
 ( 1.000000000000000000, 0.6915472827938593525, 1.000000000000000000),
 ( 1.000000000000000000, 0.6902979293261688465, 1.000000000000000000),
 ( 1.000000000000000000, 0.6865737038807442350, 1.000000000000000000),
 ( 1.000000000000000000, 0.6841432992373190913, 1.000000000000000000),
 ( 1.000000000000000000, 0.6806030716582376350, 1.000000000000000000),
 ( 1.000000000000000000, 0.6794407469212847550, 1.000000000000000000),
 ( 1.000000000000000000, 0.6771618041792656362, 1.000000000000000000),
 ( 1.000000000000000000, 0.6760782311690274327, 1.000000000000000000),
 ( 1.000000000000000000, 0.6730262767741563845, 1.000000000000000000),
 ( 1.000000000000000000, 0.6712352064082731662, 1.000000000000000000),
 ( 1.000000000000000000, 0.6689250498628499519, 1.000000000000000000),
 ( 1.000000000000000000, 0.6682166586818782950, 1.000000000000000000),
 ( 1.000000000000000000, 0.6669646655643757249, 1.000000000000000000),
 ( 1.000000000000000000, 0.6664264744289446485, 1.000000000000000000),
 ( 1.000000000000000000, 0.6650728498231318619, 1.000000000000000000),
 ( 1.000000000000000000, 0.6645102704218179834, 1.000000000000000000),
 ( 1.000000000000000000, 0.6642977373962596355, 1.000000000000000000) ) ) 
 REPRESENTATION_ITEM ( '' )  SURFACE ( )  );
#5514=CARTESIAN_POINT ( 'NONE',  ( -171.2229998886518274, 121.4597901571797252, 9.827342307218824402 ) ) ;
#5515=CARTESIAN_POINT ( 'NONE',  ( -220.6713114466640207, 151.8719187835573052, -4.501197839774258469 ) ) ;
#5525=CARTESIAN_POINT ( 'NONE',  ( -221.5359850654323282, 150.3227202646742455, -2.975602802620230580 ) ) ;
#5562=ORIENTED_EDGE ( 'NONE', *, *, #859, .T. ) ;
#5565=CARTESIAN_POINT ( 'NONE',  ( -169.9274309510963406, 128.7925441011331031, 1.515441478317341994 ) ) ;
#5569=CARTESIAN_POINT ( 'NONE',  ( -217.2107590478593977, 140.9839873040922100, -2.964974570226843742 ) ) ;
#5584=CARTESIAN_POINT ( 'NONE',  ( -179.8866491758529094, 122.3521977864031243, 9.530069280832647038 ) ) ;
#5596=CARTESIAN_POINT ( 'NONE',  ( -173.0522527676590414, 118.1823964801743188, 8.186264704042805818 ) ) ;
#5597=CARTESIAN_POINT ( 'NONE',  ( -223.0526696604661652, 147.6053417333511106, -2.589170730542551535 ) ) ;
#5604=CARTESIAN_POINT ( 'NONE',  ( -223.7665658100024189, 146.3262847186648230, -1.606151718348904689 ) ) ;
#5611=CARTESIAN_POINT ( 'NONE',  ( -198.5677679834141713, 144.7676449960911498, 2.500000000000000000 ) ) ;
#5639=CARTESIAN_POINT ( 'NONE',  ( -174.9627087613145306, 131.1742099673107305, -0.4568654681747568169 ) ) ;
#5642=CARTESIAN_POINT ( 'NONE',  ( -203.7063805325860812, 135.3711971156951677, -4.642206099735014746 ) ) ;
#5658=CARTESIAN_POINT ( 'NONE',  ( -178.4568510201948186, 124.9139056227158733, 10.12588066961104261 ) ) ;
#5670=CARTESIAN_POINT ( 'NONE',  ( -167.8411187277642114, 127.5189611227023363, 3.660767585630689602 ) ) ;
#5671=CARTESIAN_POINT ( 'NONE',  ( -219.7323164117629801, 149.4657087312641863, -4.974268084325299100 ) ) ;
#5681=DIRECTION ( 'NONE',  ( 1.000000000000000000, 0.000000000000000000, 0.000000000000000000 ) ) ;
#5699=CARTESIAN_POINT ( 'NONE',  ( -225.6574687014862661, 142.9384353668704364, 3.546568788011186690 ) ) ;
#5717=ORIENTED_EDGE ( 'NONE', *, *, #2728, .F. ) ;
#5718=CARTESIAN_POINT ( 'NONE',  ( -200.1353104204616500, 130.1171604195963880, -2.964974570226841522 ) ) ;
#5733=CARTESIAN_POINT ( 'NONE',  ( -202.2835283783994953, 137.9722283379741725, 10.16010209732750624 ) ) ;
#5743=CARTESIAN_POINT ( 'NONE',  ( -167.8000917210836747, 127.5924674453244592, 2.732326210438932979 ) ) ;
#5744=CARTESIAN_POINT ( 'NONE',  ( -223.5878110270859906, 146.6465519720144073, -4.388772443223475150 ) ) ;
#5746=CARTESIAN_POINT ( 'NONE',  ( -216.7216729069047005, 154.8463875879168086, 3.280095325655492111 ) ) ;
#5763=EDGE_LOOP ( 'NONE', ( #10608, #8550, #8030, #9795, #10279 ) ) ;
#5771=ORIENTED_EDGE ( 'NONE', *, *, #2728, .T. ) ;
#5791=CARTESIAN_POINT ( 'NONE',  ( -189.5834090937817109, 129.2672479736120010, -4.642206099735012970 ) ) ;
#5809=CARTESIAN_POINT ( 'NONE',  ( -213.9961813491638623, 134.6717504882919911, 3.478895870929492595 ) ) ;
#5819=CIRCLE ( 'NONE', #9352, 1.999999999999991118 ) ;
#5822=CARTESIAN_POINT ( 'NONE',  ( -222.9037195049596676, 147.8722093182038293, -4.873412262819154961 ) ) ;
#5823=CARTESIAN_POINT ( 'NONE',  ( -220.0428052216640538, 148.9356522631746884, 9.942732236775652765 ) ) ;
#5854=CARTESIAN_POINT ( 'NONE',  ( -224.5811800873044604, 144.8667753680074384, 1.831365460742872209 ) ) ;
#5872=CARTESIAN_POINT ( 'NONE',  ( -198.5677679834141713, 144.7676449960911498, 2.500000000000000000 ) ) ;
#5875=CARTESIAN_POINT ( 'NONE',  ( -198.4137021260360711, 129.4968702780754199, -2.964974570226842410 ) ) ;
#5889=CARTESIAN_POINT ( 'NONE',  ( -178.4228374502453107, 119.2657932277225967, 7.804961498744191317 ) ) ;
#5900=CARTESIAN_POINT ( 'NONE',  ( -221.2834769382098443, 150.7751282116832670, -2.840239297744243885 ) ) ;
#5917=CARTESIAN_POINT ( 'NONE',  ( -214.8759442515754188, 153.8597017879883424, 3.478855109513426580 ) ) ;
#5924=CARTESIAN_POINT ( 'NONE',  ( -222.6691881216298725, 143.9122218626206688, 7.777047806907320115 ) ) ;
#5931=DIRECTION ( 'NONE',  ( -0.8731965799097684000, 0.4873681696970817989, 0.000000000000000000 ) ) ;
#5948=CARTESIAN_POINT ( 'NONE',  ( -201.8614823352862970, 146.6162971164513635, 1.515441477536285220 ) ) ;
#5967=CARTESIAN_POINT ( 'NONE',  ( -214.8265656857867327, 135.2606554265309740, 1.515400478619088664 ) ) ;
#5970=CARTESIAN_POINT ( 'NONE',  ( -212.8994228580217509, 136.6308034654096559, 7.918248976830621011 ) ) ;
#5981=CARTESIAN_POINT ( 'NONE',  ( -219.0612485848473057, 150.7318302238501246, 9.479016549696966720 ) ) ;
#5986=CARTESIAN_POINT ( 'NONE',  ( -218.4444600228138711, 155.8616726660956715, 2.500000000270498735 ) ) ;
#5999=CARTESIAN_POINT ( 'NONE',  ( -167.5053995445195767, 127.4304153265770907, 2.500000001036336350 ) ) ;
#6008=CARTESIAN_POINT ( 'NONE',  ( -225.1775117427411601, 143.7983535990246651, 6.320880672221801611 ) ) ;
#6033=CARTESIAN_POINT ( 'NONE',  ( -169.4320859569187405, 123.9702250307836238, -4.722862203412457660 ) ) ;
#6050=CARTESIAN_POINT ( 'NONE',  ( -201.1640730962011219, 128.1953734590158263, 1.515400478619091773 ) ) ;
#6056=CARTESIAN_POINT ( 'NONE',  ( -200.8348121886614024, 140.6195990399117477, 9.578254705571838556 ) ) ;
#6062=CARTESIAN_POINT ( 'NONE',  ( -214.8263955852045797, 135.2609574206205991, 2.431555724346859737 ) ) ;
#6069=CARTESIAN_POINT ( 'NONE',  ( -223.3321795807909211, 142.5930735833125027, 5.590921595890676166 ) ) ;
#6092=CARTESIAN_POINT ( 'NONE',  ( -220.1303546989248048, 152.8411277130203700, 6.239059799508164694 ) ) ;
#6094=CARTESIAN_POINT ( 'NONE',  ( -222.8166798902130665, 143.6204043892651043, 7.418049566996383959 ) ) ;
#6113=CARTESIAN_POINT ( 'NONE',  ( -175.7692568323954845, 129.7291524912800185, -2.973479603620230893 ) ) ;
#6124=B_SPLINE_CURVE_WITH_KNOTS ( 'NONE', 3,
 ( #11842, #6797, #853, #15219, #11610, #6880, #5611, #1013, #10660, #10734, #2282, #2125, #4573, #15448, #3394, #773, #9395 ),
 .UNSPECIFIED., .F., .F.,
 ( 4, 2, 2, 2, 2, 2, 3, 4 ),
 ( 0.04000000000000142331, 0.2455027589669699362, 0.3041813370740077405, 0.5308033955276700855, 0.6372805264318512908, 0.8233339832829627003, 1.000000000000000000, 1.159999999999998366 ),
 .UNSPECIFIED. ) ;
#6128=CARTESIAN_POINT ( 'NONE',  ( -173.9416064256852508, 115.8726071073731987, 3.216677072105399660 ) ) ;
#6131=CARTESIAN_POINT ( 'NONE',  ( -202.2835283783994953, 137.9722283379741725, 10.16010209732750624 ) ) ;
#6136=CARTESIAN_POINT ( 'NONE',  ( -220.4645760442968481, 140.7127987834906264, 2.431555724346865510 ) ) ;
#6141=CARTESIAN_POINT ( 'NONE',  ( -224.4234439893976969, 145.1493843477977066, 0.4584262417075776752 ) ) ;
#6153=( NAMED_UNIT ( * ) PLANE_ANGLE_UNIT ( ) SI_UNIT ( $, .RADIAN. ) );
#6162=CARTESIAN_POINT ( 'NONE',  ( -187.9175675668324175, 138.8130845598205667, 3.478855109513427468 ) ) ;
#6171=CARTESIAN_POINT ( 'NONE',  ( -223.5769481064250499, 146.6660145995820130, 6.853793408916477148 ) ) ;
#6174=CARTESIAN_POINT ( 'NONE',  ( -223.6441180315265456, 146.5456691348633740, 6.731302149999042861 ) ) ;
#6194=CARTESIAN_POINT ( 'NONE',  ( -180.1141531658810777, 134.0357633396332915, -0.4547266291960706530 ) ) ;
#6208=CARTESIAN_POINT ( 'NONE',  ( -192.4489746382803048, 130.7761537121523361, -4.642206099735005864 ) ) ;
#6211=CARTESIAN_POINT ( 'NONE',  ( -174.6331699355062028, 120.3494046152724763, 9.441255307061881652 ) ) ;
#6223=CARTESIAN_POINT ( 'NONE',  ( -215.8266853215729668, 152.1588074852305112, 7.919662025281898998 ) ) ;
#6236=CARTESIAN_POINT ( 'NONE',  ( -192.1704923257120754, 141.1970532186197431, 2.500000000000000000 ) ) ;
#6240=CARTESIAN_POINT ( 'NONE',  ( -221.4549156970492163, 150.4679687638771100, 7.826104580404325439 ) ) ;
#6244=CARTESIAN_POINT ( 'NONE',  ( -224.1075752074748948, 145.7153128536473332, 5.693834061489701170 ) ) ;
#6248=CARTESIAN_POINT ( 'NONE',  ( -172.6903511823495592, 118.8307999792220642, -4.176935792781210743 ) ) ;
#6267=CARTESIAN_POINT ( 'NONE',  ( -213.3556830655219585, 148.0789703896194567, -4.640918829492433950 ) ) ;
#6282=CARTESIAN_POINT ( 'NONE',  ( -222.1045353819713455, 144.9552801561289357, -3.848506573863026414 ) ) ;
#6283=CARTESIAN_POINT ( 'NONE',  ( -173.2784152866543934, 122.7799518889917465, -5.329639836781006501 ) ) ;
#6285=CARTESIAN_POINT ( 'NONE',  ( -219.6650276661029011, 145.2909210783078890, 9.577123744044234499 ) ) ;
#6293=CARTESIAN_POINT ( 'NONE',  ( -225.4857480675195802, 143.2460998381742456, -0.09261257463428765324 ) ) ;
#6299=CARTESIAN_POINT ( 'NONE',  ( -215.0595991585972513, 153.5311831015895052, 5.434754235172610137 ) ) ;
#6318=CARTESIAN_POINT ( 'NONE',  ( -180.9926919874575333, 132.4923963613727267, 7.919662025281893669 ) ) ;
#6326=DIRECTION ( 'NONE',  ( -0.4873681696970817989, -0.8731965799097684000, 0.000000000000000000 ) ) ;
#6328=CARTESIAN_POINT ( 'NONE',  ( -216.7216729069043026, 154.8463875879177181, 3.280095325646671167 ) ) ;
#6367=CARTESIAN_POINT ( 'NONE',  ( -198.8906912147545540, 132.4339616203728838, -4.642206099735012970 ) ) ;
#6370=CARTESIAN_POINT ( 'NONE',  ( -213.7840885461983760, 135.0504928752735339, -0.4555467707853347870 ) ) ;
#6384=CARTESIAN_POINT ( 'NONE',  ( -211.3030747601025610, 151.8655312830997559, 3.478855109513426580 ) ) ;
#6399=CARTESIAN_POINT ( 'NONE',  ( -221.0074014867128369, 151.2697607195771639, -4.739390644780034023 ) ) ;
#6400=CARTESIAN_POINT ( 'NONE',  ( -212.2525635541804547, 150.1126023820536375, 7.919662025281898998 ) ) ;
#6405=CARTESIAN_POINT ( 'NONE',  ( -223.9498498189288682, 145.9979026459368470, 6.124526283558925144 ) ) ;
#6408=CARTESIAN_POINT ( 'NONE',  ( -219.5220412541523274, 149.8943906618940787, 9.781285959214518044 ) ) ;
#6430=CARTESIAN_POINT ( 'NONE',  ( -206.0179204244930702, 148.9258921110169638, 2.500000000000000000 ) ) ;
#6445=CARTESIAN_POINT ( 'NONE',  ( -194.2672495621651478, 127.5518908598051127, -0.4555467707853320669 ) ) ;
#6448=CARTESIAN_POINT ( 'NONE',  ( -201.1640730962011219, 128.1953734590158263, 3.478895870929496148 ) ) ;
#6452=ORIENTED_EDGE ( 'NONE', *, *, #10204, .T. ) ;
#6459=ORIENTED_EDGE ( 'NONE', *, *, #13028, .T. ) ;
#6475=CARTESIAN_POINT ( 'NONE',  ( -216.6908943189923207, 154.8992719724514302, 2.316389262299374252 ) ) ;
#6476=CARTESIAN_POINT ( 'NONE',  ( -194.7616377892423714, 140.1172406977107130, 7.919662025281898998 ) ) ;
#6486=CARTESIAN_POINT ( 'NONE',  ( -219.4693564985508942, 154.0254097482049929, 1.294062626359073542 ) ) ;
#6488=CARTESIAN_POINT ( 'NONE',  ( -220.8889415488412169, 151.4820002933464025, 7.400835299683578228 ) ) ;
#6490=CARTESIAN_POINT ( 'NONE',  ( -169.4759604733452250, 124.5898855086296919, -4.204736276848058729 ) ) ;
#6507=CARTESIAN_POINT ( 'NONE',  ( -192.1704923257120754, 141.1970532186197431, 2.500000000000000000 ) ) ;
#6522=CARTESIAN_POINT ( 'NONE',  ( -220.9124392735551226, 147.2477244607945579, -4.927242291365885762 ) ) ;
#6524=CARTESIAN_POINT ( 'NONE',  ( -181.1480734112017501, 126.1383063644306617, -5.230826428279600648 ) ) ;
#6527=CARTESIAN_POINT ( 'NONE',  ( -191.4964613557999655, 125.7493975051623352, 1.515400478619084224 ) ) ;
#6540=CARTESIAN_POINT ( 'NONE',  ( -219.4661802592007689, 154.0311004795854046, 7.909502539118774322 ) ) ;
#6552=B_SPLINE_CURVE_WITH_KNOTS ( 'NONE', 3,
 ( #6877, #11838, #1011, #850, #8229 ),
 .UNSPECIFIED., .F., .F.,
 ( 4, 1, 4 ),
 ( 0.02346780518444461713, 0.02385965792372440192, 0.02425151066300419017 ),
 .UNSPECIFIED. ) ;
#6554=CARTESIAN_POINT ( 'NONE',  ( -219.4360840196858646, 154.0850226169894768, 3.058976617618253346 ) ) ;
#6567=CARTESIAN_POINT ( 'NONE',  ( -219.6570823573851783, 153.6890694041141217, 4.765787677119769583 ) ) ;
#6569=CARTESIAN_POINT ( 'NONE',  ( -170.4088383823848574, 122.9184882974554256, -5.007687358117594911 ) ) ;
#6590=CARTESIAN_POINT ( 'NONE',  ( -167.5010204568278027, 127.4382611495783237, 1.515441478572621570 ) ) ;
#6603=CARTESIAN_POINT ( 'NONE',  ( -189.8662655649658859, 135.3588663075204579, -4.640918829492423292 ) ) ;
#6605=CARTESIAN_POINT ( 'NONE',  ( -214.8265656857867327, 135.2606554265309740, 1.515400478619088664 ) ) ;
#6621=CARTESIAN_POINT ( 'NONE',  ( -188.3680287392151627, 131.4989828868489781, 10.16010209732750269 ) ) ;
#6635=PRODUCT_DEFINITION ( 'UNKNOWN', '', #1721, #6785 ) ;
#6637=CARTESIAN_POINT ( 'NONE',  ( -216.9798112490933306, 154.4040521289827836, -0.4892415239726802256 ) ) ;
#6646=CARTESIAN_POINT ( 'NONE',  ( -218.7420931059136251, 151.3070553729347978, 9.190923517782497498 ) ) ;
#6684=CARTESIAN_POINT ( 'NONE',  ( -219.4290858278833980, 154.0975609761335932, -2.973479603620232226 ) ) ;
#6687=CARTESIAN_POINT ( 'NONE',  ( -214.6152097961127367, 135.6358893629490581, -0.4555467707853336767 ) ) ;
#6697=ORIENTED_EDGE ( 'NONE', *, *, #3533, .T. ) ;
#6699=CARTESIAN_POINT ( 'NONE',  ( -207.1471226269450767, 137.0919095985319132, 9.577123744044238052 ) ) ;
#6710=CARTESIAN_POINT ( 'NONE',  ( -174.2842449426172209, 115.9750891085876390, 2.645078463637116073 ) ) ;
#6711=CARTESIAN_POINT ( 'NONE',  ( -219.8521491127885383, 153.3395766914946421, -3.516840477861103320 ) ) ;
#6719=CARTESIAN_POINT ( 'NONE',  ( -220.2506544535641524, 152.6255918187081875, -1.607790317205930686 ) ) ;
#6738=CARTESIAN_POINT ( 'NONE',  ( -223.6165645121877503, 142.0072334165735981, 2.089048013359927847 ) ) ;
#6752=CARTESIAN_POINT ( 'NONE',  ( -172.3538414453648500, 130.1468270526879110, 1.515441478062062641 ) ) ;
#6755=CARTESIAN_POINT ( 'NONE',  ( -171.9831566630682858, 119.3897064310878875, -4.822481523602708542 ) ) ;
#6768=CARTESIAN_POINT ( 'NONE',  ( -208.4006302466032992, 134.8330880460140122, 7.918248976830637886 ) ) ;
#6780=CARTESIAN_POINT ( 'NONE',  ( -173.3690302610533251, 117.6148398750801789, 7.519404742434161903 ) ) ;
#6782=CARTESIAN_POINT ( 'NONE',  ( -221.5356353662852200, 150.3233468055901767, -2.966311635581158956 ) ) ;
#6785=PRODUCT_DEFINITION_CONTEXT ( 'detailed design', #713, 'design' ) ;
#6792=CARTESIAN_POINT ( 'NONE',  ( -218.4677351830674183, 155.8199715629180275, 3.280001329119076825 ) ) ;
#6797=CARTESIAN_POINT ( 'NONE',  ( -213.7073284247934453, 153.2176779349464368, 2.500000000000000000 ) ) ;
#6816=DIRECTION ( 'NONE',  ( -0.05388311488299379198, -0.09654005853512973023, 0.9938695221348423647 ) ) ;
#6828=AXIS2_PLACEMENT_3D ( 'NONE', #1342, #8546, #13258 ) ;
#6832=CARTESIAN_POINT ( 'NONE',  ( -177.3513212993587729, 132.9361332244957055, 1.515441477536284109 ) ) ;
#6836=CARTESIAN_POINT ( 'NONE',  ( -170.7063108826370694, 121.6823135672476752, -5.361935827173478941 ) ) ;
#6851=CARTESIAN_POINT ( 'NONE',  ( -222.1166800156826184, 149.2823141075699880, 10.12588066961105504 ) ) ;
#6863=CARTESIAN_POINT ( 'NONE',  ( -174.1472389072507383, 116.2205569272661734, 4.466624464644515236 ) ) ;
#6864=CARTESIAN_POINT ( 'NONE',  ( -224.4909276189729894, 145.0284768322981108, -3.162994880121249963 ) ) ;
#6877=CARTESIAN_POINT ( 'NONE',  ( -216.6980668629938123, 154.8869363267023687, 2.500000000158653091 ) ) ;
#6880=CARTESIAN_POINT ( 'NONE',  ( -201.8658614229783268, 146.6084512934502584, 2.500000000000000000 ) ) ;
#6882=CLOSED_SHELL ( 'NONE', ( #15576, #15604, #3782, #717, #4981, #8903, #6933, #1962, #7840 ) ) ;
#6909=CARTESIAN_POINT ( 'NONE',  ( -208.4264987254875052, 144.6230976266233483, -4.640918829492436615 ) ) ;
#6912=CARTESIAN_POINT ( 'NONE',  ( -204.9433645127610646, 133.1096489332827275, -2.964974570226844186 ) ) ;
#6924=( NAMED_UNIT ( * ) SI_UNIT ( $, .STERADIAN. ) SOLID_ANGLE_UNIT ( ) );
#6931=CARTESIAN_POINT ( 'NONE',  ( -169.4720549176639395, 123.8986143635366943, 9.496311331651778431 ) ) ;
#6933=ADVANCED_FACE ( 'NONE', ( #8997 ), #5512, .T. ) ;
#6942=CARTESIAN_POINT ( 'NONE',  ( -171.8875587097026028, 120.2691287111299374, 9.563504314567204290 ) ) ;
#6943=CARTESIAN_POINT ( 'NONE',  ( -220.9930168758324669, 147.0937147668695957, -4.878251604516314899 ) ) ;
#6944=CARTESIAN_POINT ( 'NONE',  ( -223.6175992062213140, 142.0096542461538718, 2.866221285019154852 ) ) ;
#6991=CARTESIAN_POINT ( 'NONE',  ( -175.7369819406991382, 118.3688719364822646, -3.133266157129962259 ) ) ;
#7003=CARTESIAN_POINT ( 'NONE',  ( -179.3772030532177837, 117.5545944912402661, 1.382365641875445528 ) ) ;
#7014=CARTESIAN_POINT ( 'NONE',  ( -223.9433292823694046, 146.0095852107350254, -1.211090774047295371 ) ) ;
#7025=CARTESIAN_POINT ( 'NONE',  ( -174.7846310273254176, 131.4932641812416421, 2.500000000270498735 ) ) ;
#7046=CARTESIAN_POINT ( 'NONE',  ( -225.6712625649270478, 142.9137214952622514, 1.583163137451349511 ) ) ;
#7054=CARTESIAN_POINT ( 'NONE',  ( -222.0995690897443922, 149.3129710173510887, 2.431557144026069928 ) ) ;
#7069=CARTESIAN_POINT ( 'NONE',  ( -212.3935931674892856, 139.5852744332111683, -4.642206099735020963 ) ) ;
#7073=EDGE_CURVE ( 'NONE', #14472, #9526, #14622, .T. ) ;
#7085=CARTESIAN_POINT ( 'NONE',  ( -223.5244451892836537, 142.1828519274101836, 0.6844914428394093253 ) ) ;
#7086=CARTESIAN_POINT ( 'NONE',  ( -209.4369489341841586, 132.9646294043573675, 1.515400478619103763 ) ) ;
#7098=CARTESIAN_POINT ( 'NONE',  ( -224.1994838851412624, 145.5506440303793454, -0.5027386706791425741 ) ) ;
#7099=CARTESIAN_POINT ( 'NONE',  ( -218.7472433255651936, 151.2978141277262409, 9.195915456466519089 ) ) ;
#7118=CARTESIAN_POINT ( 'NONE',  ( -211.2987210398670186, 151.8733316563206586, 2.500000000000000000 ) ) ;
#7130=CARTESIAN_POINT ( 'NONE',  ( -224.5263272834600059, 144.9650527765320192, 3.765861206744722356 ) ) ;
#7145=CARTESIAN_POINT ( 'NONE',  ( -177.3557003870508595, 132.9282874014947140, 2.500000000000000000 ) ) ;
#7149=CARTESIAN_POINT ( 'NONE',  ( -206.8675068987516283, 149.4103724542255804, 1.515441477536285220 ) ) ;
#7168=CARTESIAN_POINT ( 'NONE',  ( -225.5658467874630446, 143.1025904080742919, 5.367833425961707761 ) ) ;
#7171=CARTESIAN_POINT ( 'NONE',  ( -216.0863581598438543, 143.0557482234525253, 9.577123744044239828 ) ) ;
#7184=CARTESIAN_POINT ( 'NONE',  ( -221.9362923240670114, 145.3446861235061931, 9.019126511735166218 ) ) ;
#7208=ORIENTED_EDGE ( 'NONE', *, *, #765, .F. ) ;
#7209=CARTESIAN_POINT ( 'NONE',  ( -222.1550322922110752, 144.9192006534358370, 8.707947314692312091 ) ) ;
#7231=CARTESIAN_POINT ( 'NONE',  ( -192.1661132380199604, 141.2048990416207630, 1.515441477536284332 ) ) ;
#7239=SURFACE_SIDE_STYLE ('',( #897 ) ) ;
#7245=CARTESIAN_POINT ( 'NONE',  ( -187.5349220100912930, 120.9938564418671518, 1.515400478619096658 ) ) ;
#7248=CARTESIAN_POINT ( 'NONE',  ( -169.4720549176639395, 123.8986143635366943, 9.496311331651778431 ) ) ;
#7258=CARTESIAN_POINT ( 'NONE',  ( -217.3694051724266671, 153.7302547217275333, 6.764857390201539644 ) ) ;
#7282=CARTESIAN_POINT ( 'NONE',  ( -223.3638075659000606, 147.0478893353539718, 7.150006577359191873 ) ) ;
#7303=CARTESIAN_POINT ( 'NONE',  ( -200.7948432279144129, 140.6912097071583787, -4.640918829492429509 ) ) ;
#7320=CARTESIAN_POINT ( 'NONE',  ( -182.0950013669840359, 118.3955881831737997, 1.446957622915671537 ) ) ;
#7324=CARTESIAN_POINT ( 'NONE',  ( -173.3126422121597443, 122.7186289792270912, 10.06128868882609062 ) ) ;
#7354=CARTESIAN_POINT ( 'NONE',  ( -193.7244371550166022, 142.0541455854551600, 3.478855109513427468 ) ) ;
#7362=CARTESIAN_POINT ( 'NONE',  ( -225.6149816284549559, 143.0145576275852193, 4.031212713769876999 ) ) ;
#7384=CARTESIAN_POINT ( 'NONE',  ( -215.0356418556126812, 153.5741063705486908, -0.4547266291960771478 ) ) ;
#7400=CARTESIAN_POINT ( 'NONE',  ( -188.3338018137096128, 131.5603057966125675, -5.230826428279604201 ) ) ;
#7403=CARTESIAN_POINT ( 'NONE',  ( -182.2596580518439850, 130.2653702959948987, 9.578254705571840333 ) ) ;
#7434=FACE_OUTER_BOUND ( 'NONE', #5010, .T. ) ;
#7436=CARTESIAN_POINT ( 'NONE',  ( -222.2306213242449360, 149.0781703675127403, 7.930418395707709678 ) ) ;
#7438=CARTESIAN_POINT ( 'NONE',  ( -168.9408230362998893, 125.5486682295035905, -3.359583683245268126 ) ) ;
#7447=SHAPE_DEFINITION_REPRESENTATION ( #12800, #13652 ) ;
#7448=EDGE_LOOP ( 'NONE', ( #5144, #5562 ) ) ;
#7456=CARTESIAN_POINT ( 'NONE',  ( -180.9555975561403613, 132.5588568579215973, -2.963320117457099112 ) ) ;
#7469=CARTESIAN_POINT ( 'NONE',  ( -218.9522465171050953, 150.9009417352626770, -4.531563180531605006 ) ) ;
#7470=CARTESIAN_POINT ( 'NONE',  ( -174.6098962832414827, 120.3911030166530054, -4.778074536717329401 ) ) ;
#7473=CARTESIAN_POINT ( 'NONE',  ( -183.7478807014743722, 127.6480629723144347, 10.16010209732750624 ) ) ;
#7481=CARTESIAN_POINT ( 'NONE',  ( -225.2945142095777840, 143.5887253133888635, -1.007486474111332075 ) ) ;
#7485=CARTESIAN_POINT ( 'NONE',  ( -192.3703904092303105, 140.8200239622036918, 5.434754235172604808 ) ) ;
#7502=CARTESIAN_POINT ( 'NONE',  ( -186.0759242617834559, 135.7072545306847076, 7.919662025281895446 ) ) ;
#7507=CARTESIAN_POINT ( 'NONE',  ( -219.4360840196855804, 154.0850226169901305, 3.058976617611859794 ) ) ;
#7509=CARTESIAN_POINT ( 'NONE',  ( -218.5426395586106025, 155.6857686161635286, 4.229107391422298967 ) ) ;
#7549=CARTESIAN_POINT ( 'NONE',  ( -217.2107590478593977, 140.9839873040922100, -2.964974570226843742 ) ) ;
#7552=CARTESIAN_POINT ( 'NONE',  ( -209.4369489341841586, 132.9646294043573675, 3.478895870929508582 ) ) ;
#7561=DIRECTION ( 'NONE',  ( 0.4873681696970831312, 0.8731965799097676229, 0.000000000000000000 ) ) ;
#7565=CARTESIAN_POINT ( 'NONE',  ( -173.3366878899875019, 128.3846004176512849, 7.899914667150486736 ) ) ;
#7582=CARTESIAN_POINT ( 'NONE',  ( -180.1381104688653920, 133.9928400706745037, 5.434754235172599479 ) ) ;
#7590=CARTESIAN_POINT ( 'NONE',  ( -219.4552112669440191, 154.0507531510554884, 3.411777084580434938 ) ) ;
#7592=CARTESIAN_POINT ( 'NONE',  ( -218.6814998127593412, 155.4369786734033880, 5.141710482893284251 ) ) ;
#7629=CARTESIAN_POINT ( 'NONE',  ( -217.1265240672488233, 154.1501268790366339, -1.115935190456407433 ) ) ;
#7630=CARTESIAN_POINT ( 'NONE',  ( -181.9037801448002938, 118.7381910193847716, -0.5218507872395746761 ) ) ;
#7633=CARTESIAN_POINT ( 'NONE',  ( -221.7331157600676192, 141.5908957077777188, 3.478895870929496148 ) ) ;
#7636=ORIENTED_EDGE ( 'NONE', *, *, #8600, .T. ) ;
#7647=CARTESIAN_POINT ( 'NONE',  ( -180.1381104688653920, 133.9928400706745037, 5.434754235172599479 ) ) ;
#7659=CARTESIAN_POINT ( 'NONE',  ( -218.7271737403003442, 151.3100222557285122, -4.321910846754870583 ) ) ;
#7660=CARTESIAN_POINT ( 'NONE',  ( -199.6024142766798946, 142.8729305612646385, 7.919662025281897222 ) ) ;
#7668=CARTESIAN_POINT ( 'NONE',  ( -222.1421115826539392, 149.2367494632589455, 7.942719255002825385 ) ) ;
#7672=CARTESIAN_POINT ( 'NONE',  ( -221.4749990704029301, 150.4319862478757273, 9.846583645253028649 ) ) ;
#7674=CARTESIAN_POINT ( 'NONE',  ( -170.0824065865490979, 123.5033421008434686, -4.824223088519030256 ) ) ;
#7693=CARTESIAN_POINT ( 'NONE',  ( -174.7846310273254176, 131.4932641812416421, 2.500000000270498735 ) ) ;
#7710=CARTESIAN_POINT ( 'NONE',  ( -219.4863873870018267, 149.9206971141745441, -4.874325179114736173 ) ) ;
#7711=CARTESIAN_POINT ( 'NONE',  ( -212.8881127827856687, 136.6510672405775892, -2.964974570226852624 ) ) ;
#7714=CARTESIAN_POINT ( 'NONE',  ( -221.7331157600676192, 141.5908957077777188, 1.515400478619091551 ) ) ;
#7727=CARTESIAN_POINT ( 'NONE',  ( -185.2098801967860595, 137.3018090142982146, 3.478855109513427468 ) ) ;
#7741=CARTESIAN_POINT ( 'NONE',  ( -217.3145496446415450, 153.8230492215183176, -1.760001856877286608 ) ) ;
#7748=CARTESIAN_POINT ( 'NONE',  ( -224.4234439893150181, 145.1493843479457553, 0.4584262417508254694 ) ) ;
#7751=CARTESIAN_POINT ( 'NONE',  ( -218.9392864022120193, 154.9751135327425970, 6.220092860173763505 ) ) ;
#7786=CARTESIAN_POINT ( 'NONE',  ( -211.2943419521749888, 151.8811774793218490, 1.515441477536285220 ) ) ;
#7790=CARTESIAN_POINT ( 'NONE',  ( -183.9313806081839289, 121.1548445249323720, 7.918248976830652097 ) ) ;
#7805=CARTESIAN_POINT ( 'NONE',  ( -205.6684400016210645, 139.7560197894119085, 10.16010209732751157 ) ) ;
#7819=CARTESIAN_POINT ( 'NONE',  ( -218.9290471127720821, 154.9934588271201505, -1.343261102213330949 ) ) ;
#7832=CARTESIAN_POINT ( 'NONE',  ( -219.0004266419835801, 154.8655711957941890, 6.428065963712064956 ) ) ;
#7840=ADVANCED_FACE ( 'NONE', ( #4916 ), #8406, .T. ) ;
#7854=CARTESIAN_POINT ( 'NONE',  ( -206.8718859864436581, 149.4025266312245037, 2.500000000000000000 ) ) ;
#7870=CARTESIAN_POINT ( 'NONE',  ( -182.2196890910978482, 130.3369809632412739, -4.640918829492416187 ) ) ;
#7873=CARTESIAN_POINT ( 'NONE',  ( -221.5559209476002991, 141.9078401207188449, -0.4555467707853290138 ) ) ;
#7886=CARTESIAN_POINT ( 'NONE',  ( -210.8662606591548752, 142.3010704693858486, 10.16010209732750624 ) ) ;
#7897=CARTESIAN_POINT ( 'NONE',  ( -167.8991350591905416, 127.4150157579244080, 4.345048324134917372 ) ) ;
#7898=CARTESIAN_POINT ( 'NONE',  ( -216.7281194157721131, 154.8360440772405866, 1.364217605950574397 ) ) ;
#7908=CARTESIAN_POINT ( 'NONE',  ( -220.0724991394543224, 152.9447850296022864, -1.223998976589070864 ) ) ;
#7944=CARTESIAN_POINT ( 'NONE',  ( -185.2011473888584874, 137.3174552105199666, 1.515441477536283887 ) ) ;
#7948=CARTESIAN_POINT ( 'NONE',  ( -193.5420962672365022, 128.8371742780315969, -2.964974570226833084 ) ) ;
#7959=CARTESIAN_POINT ( 'NONE',  ( -198.9139648670198994, 132.3922632189928095, 9.577123744044227394 ) ) ;
#7971=CARTESIAN_POINT ( 'NONE',  ( -170.2135745989010047, 123.2683340168104422, 9.619678501396277781 ) ) ;
#7972=CARTESIAN_POINT ( 'NONE',  ( -219.2752461992650979, 150.3093291563185687, -4.757798792355696804 ) ) ;
#7981=CARTESIAN_POINT ( 'NONE',  ( -223.0548572358123067, 147.6014223487273682, -2.597100425689188086 ) ) ;
#8006=CARTESIAN_POINT ( 'NONE',  ( -174.2824251065520968, 115.9783496305641535, 2.177446462082195389 ) ) ;
#8007=CARTESIAN_POINT ( 'NONE',  ( -223.5918188539070002, 142.0538562971642307, 1.612306317632525854 ) ) ;
#8018=CARTESIAN_POINT ( 'NONE',  ( -174.4670243326416994, 126.3579851466298010, -4.682492215613329734 ) ) ;
#8021=CARTESIAN_POINT ( 'NONE',  ( -205.6342130761154863, 139.8173426991758959, -5.230826428279590878 ) ) ;
#8030=ORIENTED_EDGE ( 'NONE', *, *, #11962, .F. ) ;
#8037=CARTESIAN_POINT ( 'NONE',  ( -196.0016709267559349, 137.8086561579936813, 9.578254705571842109 ) ) ;
#8040=PRODUCT ( 'Handle Grip', 'Handle Grip', '', ( #8864 ) ) ;
#8051=CARTESIAN_POINT ( 'NONE',  ( -171.5607450841399384, 120.8546666224106048, 9.733687684402502427 ) ) ;
#8052=CARTESIAN_POINT ( 'NONE',  ( -222.8126188176429991, 148.0354304998946589, -2.784116551314819610 ) ) ;
#8060=CARTESIAN_POINT ( 'NONE',  ( -224.5272311398514091, 144.9634333759256322, 1.130582765413566282 ) ) ;
#8086=CARTESIAN_POINT ( 'NONE',  ( -224.5839432122867834, 144.8618247958639245, 3.066209503615932697 ) ) ;
#8106=CARTESIAN_POINT ( 'NONE',  ( -200.7948432279144129, 140.6912097071583787, -4.640918829492429509 ) ) ;
#8110=CARTESIAN_POINT ( 'NONE',  ( -184.7739606708014719, 119.6463200498024548, -0.4555467707853387282 ) ) ;
#8122=CARTESIAN_POINT ( 'NONE',  ( -173.3126422121597443, 122.7186289792270912, 10.06128868882609062 ) ) ;
#8136=CARTESIAN_POINT ( 'NONE',  ( -173.7035685021366476, 117.0154621025335899, 6.591438069051481996 ) ) ;
#8137=CARTESIAN_POINT ( 'NONE',  ( -220.7684332601648407, 147.5206264611648805, -4.971276815939039473 ) ) ;
#8147=DIRECTION ( 'NONE',  ( 0.000000000000000000, 0.000000000000000000, 1.000000000000000000 ) ) ;
#8167=CARTESIAN_POINT ( 'NONE',  ( -225.6729109059797338, 142.9107682335207983, 3.303491872377302574 ) ) ;
#8182=CARTESIAN_POINT ( 'NONE',  ( -169.9318100387881714, 128.7846982781319412, 2.500000000781056997 ) ) ;
#8185=CARTESIAN_POINT ( 'NONE',  ( -211.5558396979514839, 139.0314540006070274, -4.642206099735020963 ) ) ;
#8204=CARTESIAN_POINT ( 'NONE',  ( -205.9652191273047777, 131.2378527988410326, 3.478895870929496148 ) ) ;
#8216=CARTESIAN_POINT ( 'NONE',  ( -222.7110019469168662, 143.7735985160120151, -2.692100231736752391 ) ) ;
#8217=CARTESIAN_POINT ( 'NONE',  ( -217.0204816151944840, 154.3338338561956391, 5.540248425174711500 ) ) ;
#8218=CARTESIAN_POINT ( 'NONE',  ( -216.6980668629938123, 154.8869363267023687, 2.500000000158653091 ) ) ;
#8229=CARTESIAN_POINT ( 'NONE',  ( -216.7216729069047005, 154.8463875879168086, 3.280095325655492111 ) ) ;
#8241=FACE_OUTER_BOUND ( 'NONE', #11230, .T. ) ;
#8256=CARTESIAN_POINT ( 'NONE',  ( -187.9132138465967898, 138.8208849330412988, 2.500000000000000000 ) ) ;
#8259=CARTESIAN_POINT ( 'NONE',  ( -185.2102393155530535, 125.0770951282925409, -4.642206099734998759 ) ) ;
#8273=CARTESIAN_POINT ( 'NONE',  ( -176.6594047394515314, 116.7136007993067324, 1.317773660835219740 ) ) ;
#8285=CARTESIAN_POINT ( 'NONE',  ( -224.1052059540971584, 145.7195577429836817, -0.7975646621416776494 ) ) ;
#8287=CARTESIAN_POINT ( 'NONE',  ( -222.8281890163352159, 143.5973427195760905, 7.369092821369231494 ) ) ;
#8314=CARTESIAN_POINT ( 'NONE',  ( -225.2374285875299620, 143.6910031662873735, 6.106889910990925152 ) ) ;
#8335=CARTESIAN_POINT ( 'NONE',  ( -176.9844935205031504, 127.5518652045528825, -4.662307221713766658 ) ) ;
#8353=CARTESIAN_POINT ( 'NONE',  ( -187.5349220100912930, 120.9938564418671518, 3.478895870929501921 ) ) ;
#8366=CARTESIAN_POINT ( 'NONE',  ( -221.4260126471363037, 146.2653786650752181, -4.596864862611049318 ) ) ;
#8367=CARTESIAN_POINT ( 'NONE',  ( -220.2684726731945943, 148.5160382146572999, 9.961107950553353518 ) ) ;
#8387=CARTESIAN_POINT ( 'NONE',  ( -206.0179204244930702, 148.9258921110169638, 2.500000000000000000 ) ) ;
#8398=CARTESIAN_POINT ( 'NONE',  ( -222.4225350102570928, 144.3966517966595973, 8.264308561663218811 ) ) ;
#8406=PLANE ( 'NONE',  #14430 ) ;
#8417=CARTESIAN_POINT ( 'NONE',  ( -215.7895908902557380, 152.2252679817794956, -2.963320117457100444 ) ) ;
#8426=FILL_AREA_STYLE ('',( #15495 ) ) ;
#8433=CARTESIAN_POINT ( 'NONE',  ( -213.7863261933728154, 135.0464837791089963, 5.434137442415932995 ) ) ;
#8436=CARTESIAN_POINT ( 'NONE',  ( -195.8085210632896178, 134.3768662836672547, 10.16010209732750269 ) ) ;
#8440=CARTESIAN_POINT ( 'NONE',  ( -176.8865658880463343, 116.7841877362952943, 2.239335837349317071 ) ) ;
#8444=CARTESIAN_POINT ( 'NONE',  ( -223.4286909205997063, 142.3693733871445488, -0.01250108018631108930 ) ) ;
#8446=CARTESIAN_POINT ( 'NONE',  ( -221.6474553585480578, 145.9023062856681179, 9.325220120579155392 ) ) ;
#8461=CARTESIAN_POINT ( 'NONE',  ( -172.3582205330567945, 130.1389812296867774, 2.500000000525777644 ) ) ;
#8468=ORIENTED_EDGE ( 'NONE', *, *, #9650, .F. ) ;
#8469=CARTESIAN_POINT ( 'NONE',  ( -225.0466868817139812, 144.0327468735696073, 6.738601623737560331 ) ) ;
#8477=FACE_OUTER_BOUND ( 'NONE', #14987, .T. ) ;
#8491=CARTESIAN_POINT ( 'NONE',  ( -193.7157043470890301, 142.0697917816768836, 1.515441477536284332 ) ) ;
#8499=VERTEX_POINT ( 'NONE', #3209 ) ;
#8504=CARTESIAN_POINT ( 'NONE',  ( -209.2375803003894532, 133.3242992996629539, -0.4555467707853204096 ) ) ;
#8507=CARTESIAN_POINT ( 'NONE',  ( -218.3193879687431433, 147.6986783750013217, 10.16010209732750980 ) ) ;
#8511=CARTESIAN_POINT ( 'NONE',  ( -179.4907066695405717, 117.5900258420264350, 2.301225212616437865 ) ) ;
#8516=CARTESIAN_POINT ( 'NONE',  ( -225.5942063258246719, 143.0517798435176360, 0.6110505370848023921 ) ) ;
#8526=DIRECTION ( 'NONE',  ( 0.4873681696970831312, 0.8731965799097676229, 0.000000000000000000 ) ) ;
#8539=CARTESIAN_POINT ( 'NONE',  ( -220.9079605857687341, 147.3142607384192786, 9.825007490950982358 ) ) ;
#8546=DIRECTION ( 'NONE',  ( 0.8731965799097684000, -0.4873681696970819655, -0.000000000000000000 ) ) ;
#8550=ORIENTED_EDGE ( 'NONE', *, *, #10204, .F. ) ;
#8560=CARTESIAN_POINT ( 'NONE',  ( -218.6225377568032684, 155.5426184521650441, -0.4568654681747655322 ) ) ;
#8579=CARTESIAN_POINT ( 'NONE',  ( -203.7063805325860812, 135.3711971156951677, -4.642206099735014746 ) ) ;
#8583=CARTESIAN_POINT ( 'NONE',  ( -205.6684400016210645, 139.7560197894119085, 10.16010209732751157 ) ) ;
#8587=CARTESIAN_POINT ( 'NONE',  ( -199.4123279565619100, 127.6180083311870845, 2.431555724346860181 ) ) ;
#8592=CARTESIAN_POINT ( 'NONE',  ( -223.5918188539070002, 142.0538562971642307, 1.612306317632525410 ) ) ;
#8600=EDGE_CURVE ( 'NONE', #1731, #4058, #12735, .T. ) ;
#8614=CARTESIAN_POINT ( 'NONE',  ( -219.9178674059391199, 153.2218320532828386, 5.684947844236139858 ) ) ;
#8616=CARTESIAN_POINT ( 'NONE',  ( -223.9524810574280593, 145.9931883691309622, 6.118258866120367401 ) ) ;
#8630=AXIS2_PLACEMENT_3D ( 'NONE', #12385, #9794, #6326 ) ;
#8638=CARTESIAN_POINT ( 'NONE',  ( -170.0916760340589349, 128.4977246429275226, -0.4609024664951656969 ) ) ;
#8654=CARTESIAN_POINT ( 'NONE',  ( -208.3893201713671033, 134.8533518211819739, -2.964974570226836192 ) ) ;
#8659=CARTESIAN_POINT ( 'NONE',  ( -177.0244624812495999, 127.4802545373068767, 9.556866313350486308 ) ) ;
#8674=CARTESIAN_POINT ( 'NONE',  ( -180.9926919874575333, 132.4923963613727267, 7.919662025281893669 ) ) ;
#8687=CARTESIAN_POINT ( 'NONE',  ( -193.1820620331849341, 139.2949851078578831, 7.919662025281897222 ) ) ;
#8694=CARTESIAN_POINT ( 'NONE',  ( -220.2512114020426850, 152.6245939580821300, 6.492172721524804402 ) ) ;
#8696=CARTESIAN_POINT ( 'NONE',  ( -220.1311302832748424, 152.8397381319110480, 6.240814112616865472 ) ) ;
#8698=CARTESIAN_POINT ( 'NONE',  ( -167.9692492009162663, 127.2893952669590902, -0.01570012775376914554 ) ) ;
#8728=CARTESIAN_POINT ( 'NONE',  ( -216.8024222916085932, 154.7089832689310640, 0.6433992783599493670 ) ) ;
#8729=CARTESIAN_POINT ( 'NONE',  ( -175.8505196906716890, 123.8775902107358036, -5.297343846388533173 ) ) ;
#8732=CARTESIAN_POINT ( 'NONE',  ( -191.3393351389284192, 126.0399454915928317, 5.434137442415923225 ) ) ;
#8745=CARTESIAN_POINT ( 'NONE',  ( -202.9262818645171649, 144.6968105762408072, 7.919662025281898998 ) ) ;
#8758=CARTESIAN_POINT ( 'NONE',  ( -174.9866660642990155, 131.1312866983521701, 5.432615396193912538 ) ) ;
#8764=CARTESIAN_POINT ( 'NONE',  ( -220.5182597048680577, 152.1461350040581806, 6.948896239284471754 ) ) ;
#8766=CARTESIAN_POINT ( 'NONE',  ( -218.7722506038294341, 155.2743843858097534, 5.584835994200316733 ) ) ;
#8805=CARTESIAN_POINT ( 'NONE',  ( -222.2781198963554061, 144.6180712093748753, -3.576421514447124750 ) ) ;
#8806=CARTESIAN_POINT ( 'NONE',  ( -210.8320337336493822, 142.3623933791497791, -5.230826428279598872 ) ) ;
#8809=CARTESIAN_POINT ( 'NONE',  ( -218.1518098834511648, 139.2461763302102327, 3.478895870929506362 ) ) ;
#8823=CARTESIAN_POINT ( 'NONE',  ( -172.3625742532922800, 130.1311808564658747, 3.478855110039204224 ) ) ;
#8840=CARTESIAN_POINT ( 'NONE',  ( -167.6801169734147265, 127.1165587117766336, 5.426559898713293251 ) ) ;
#8850=CARTESIAN_POINT ( 'NONE',  ( -221.9718704697112059, 149.5417631404425265, 7.948023732481154013 ) ) ;
#8864=PRODUCT_CONTEXT ( 'NONE', #9917, 'mechanical' ) ;
#8892=CARTESIAN_POINT ( 'NONE',  ( -199.2233958860587961, 127.9753750774359276, -0.4555467707853375070 ) ) ;
#8895=CARTESIAN_POINT ( 'NONE',  ( -200.9709139173866959, 128.5579952147370761, 5.434137442415933883 ) ) ;
#8903=ADVANCED_FACE ( 'NONE', ( #15517 ), #5503, .T. ) ;
#8920=CARTESIAN_POINT ( 'NONE',  ( -220.0433514299955391, 152.9970077265409998, -3.801945250988365110 ) ) ;
#8928=CARTESIAN_POINT ( 'NONE',  ( -222.3946175954399678, 148.7843453045948650, -2.994737442266849570 ) ) ;
#8931=CARTESIAN_POINT ( 'NONE',  ( -217.4665255590759614, 153.5614479664741054, 7.035142701686511124 ) ) ;
#8933=CARTESIAN_POINT ( 'NONE',  ( -171.5341366638640466, 120.9023397841524883, -5.092521039015617923 ) ) ;
#8970=CARTESIAN_POINT ( 'NONE',  ( -170.0916760340589349, 128.4977246429275226, -0.4609024664951656969 ) ) ;
#8973=CARTESIAN_POINT ( 'NONE',  ( -181.9060177919747048, 118.7341819232202909, 5.367833425961690885 ) ) ;
#8975=ORIENTED_EDGE ( 'NONE', *, *, #3132, .F. ) ;
#8996=DIRECTION ( 'NONE',  ( 0.8731965799097682890, -0.4873681696970819099, 0.000000000000000000 ) ) ;
#8997=FACE_OUTER_BOUND ( 'NONE', #5763, .T. ) ;
#9006=CARTESIAN_POINT ( 'NONE',  ( -218.4940076538873939, 155.7729003073443437, 3.755297502929312969 ) ) ;
#9018=AXIS2_PLACEMENT_3D ( 'NONE', #4157, #8996, #13789 ) ;
#9030=VERTEX_POINT ( 'NONE', #9426 ) ;
#9042=CARTESIAN_POINT ( 'NONE',  ( -179.6520503532206021, 128.8169225571170102, -4.640918829492417075 ) ) ;
#9045=CARTESIAN_POINT ( 'NONE',  ( -184.9748306402843809, 119.2867206268225999, 3.478895870929497036 ) ) ;
#9048=EDGE_CURVE ( 'NONE', #14876, #9030, #5819, .T. ) ;
#9059=CARTESIAN_POINT ( 'NONE',  ( -177.2599095556795419, 121.3508012008377932, 9.485662293947264345 ) ) ;
#9072=CARTESIAN_POINT ( 'NONE',  ( -171.3372721184446164, 121.2550535197920851, 9.804730088504793883 ) ) ;
#9124=CARTESIAN_POINT ( 'NONE',  ( -178.3861577417919477, 131.0834419243807076, -2.963320117457100888 ) ) ;
#9127=CARTESIAN_POINT ( 'NONE',  ( -173.7777028115792177, 116.1670890754947152, -0.7095712321138001322 ) ) ;
#9143=CARTESIAN_POINT ( 'NONE',  ( -209.3130641152695830, 145.0632059852189570, 9.578254705571840333 ) ) ;
#9156=CARTESIAN_POINT ( 'NONE',  ( -217.6093082865582460, 153.3060710425520199, -2.530008684083509873 ) ) ;
#9165=CARTESIAN_POINT ( 'NONE',  ( -222.5645123348136281, 148.4799522100312572, -2.927675643254317173 ) ) ;
#9177=ORIENTED_EDGE ( 'NONE', *, *, #7073, .T. ) ;
#9184=CARTESIAN_POINT ( 'NONE',  ( -225.7021444021470415, 142.8583918362506608, 2.570299564593518937 ) ) ;
#9201=CARTESIAN_POINT ( 'NONE',  ( -188.0666105031049824, 138.5497687542270739, -0.4547266291960739282 ) ) ;
#9204=CARTESIAN_POINT ( 'NONE',  ( -178.4226240946890130, 124.9752285324798606, -5.265047855996060733 ) ) ;
#9215=CARTESIAN_POINT ( 'NONE',  ( -200.1466204956978459, 130.0968966444285968, 7.918248976830634334 ) ) ;
#9227=CARTESIAN_POINT ( 'NONE',  ( -168.1084462739055425, 127.0400018604442636, 5.672933193154669596 ) ) ;
#9228=CARTESIAN_POINT ( 'NONE',  ( -224.3995683171452242, 145.1921613625067096, -3.326444132835047807 ) ) ;
#9235=CARTESIAN_POINT ( 'NONE',  ( -219.8602732323815587, 153.3250210559709217, -0.6604898276721635764 ) ) ;
#9240=CARTESIAN_POINT ( 'NONE',  ( -174.2824251065520968, 115.9783496305641535, 2.177446462082195389 ) ) ;
#9275=CARTESIAN_POINT ( 'NONE',  ( -193.9023367725753815, 141.7188637290702502, -0.4547266291960752049 ) ) ;
#9278=CARTESIAN_POINT ( 'NONE',  ( -191.1563096742665380, 133.0698578461479826, -5.230826428279597984 ) ) ;
#9290=CARTESIAN_POINT ( 'NONE',  ( -204.1871669930114024, 142.4247710585700020, 9.578254705571842109 ) ) ;
#9305=CARTESIAN_POINT ( 'NONE',  ( -221.4728790919188270, 150.4357845221465482, -4.967023597482887354 ) ) ;
#9352=AXIS2_PLACEMENT_3D ( 'NONE', #10850, #14225, #3422 ) ;
#9355=CARTESIAN_POINT ( 'NONE',  ( -174.6098962832414827, 120.3911030166530054, -4.778074536717329401 ) ) ;
#9371=CARTESIAN_POINT ( 'NONE',  ( -187.3366327499677197, 121.3409432500951937, 5.434137442415932107 ) ) ;
#9383=CARTESIAN_POINT ( 'NONE',  ( -223.1352769555567193, 147.4573377970056072, -4.744530085462122848 ) ) ;
#9384=CARTESIAN_POINT ( 'NONE',  ( -223.0197145437652466, 143.2174277694208513, 6.812014755452646675 ) ) ;
#9395=CARTESIAN_POINT ( 'NONE',  ( -167.7990583880505824, 127.5943188236592363, 2.500000001005440620 ) ) ;
#9426=CARTESIAN_POINT ( 'NONE',  ( -224.5811800873043182, 144.8667753680073531, 1.831365460742872209 ) ) ;
#9429=CARTESIAN_POINT ( 'NONE',  ( -202.2493014528935475, 138.0335512477381883, -5.230826428279597096 ) ) ;
#9449=CARTESIAN_POINT ( 'NONE',  ( -214.6174474432871762, 135.6318802667844921, 5.434137442415934771 ) ) ;
#9461=CARTESIAN_POINT ( 'NONE',  ( -221.1031640812056764, 146.8836531993028132, -4.819768081029505602 ) ) ;
#9466=CARTESIAN_POINT ( 'NONE',  ( -167.5053995445195767, 127.4304153265770907, 2.500000001036336350 ) ) ;
#9477=VECTOR ( 'NONE', #13992, 1000.000000000000114 ) ;
#9488=CARTESIAN_POINT ( 'NONE',  ( -220.3531759299249302, 148.3382346779569616, 2.431557144026069928 ) ) ;
#9507=CARTESIAN_POINT ( 'NONE',  ( -198.7485669925355012, 144.4350871509360559, -0.4547266291960735951 ) ) ;
#9509=VERTEX_POINT ( 'NONE', #4783 ) ;
#9519=CARTESIAN_POINT ( 'NONE',  ( -184.7761983179757976, 119.6423109536379883, 5.434137442415926778 ) ) ;
#9526=VERTEX_POINT ( 'NONE', #2578 ) ;
#9527=CARTESIAN_POINT ( 'NONE',  ( -209.4367884691887980, 132.9649188877714607, 2.431555724346876168 ) ) ;
#9532=CARTESIAN_POINT ( 'NONE',  ( -222.0356587614904811, 145.0888860198141685, -3.948294122849004051 ) ) ;
#9552=CARTESIAN_POINT ( 'NONE',  ( -169.9318100387881714, 128.7846982781319412, 2.500000000781056997 ) ) ;
#9561=CARTESIAN_POINT ( 'NONE',  ( -223.9066929173374376, 146.0752250096516605, 8.917334695103006581 ) ) ;
#9564=ORIENTED_EDGE ( 'NONE', *, *, #4283, .T. ) ;
#9584=CARTESIAN_POINT ( 'NONE',  ( -198.5633888957220563, 144.7754908190922549, 1.515441477536285442 ) ) ;
#9603=CARTESIAN_POINT ( 'NONE',  ( -194.4337897068680547, 127.2572260587109554, 1.515400478619095992 ) ) ;
#9606=CARTESIAN_POINT ( 'NONE',  ( -217.2220691230952525, 140.9637235289241062, 7.918248976830628116 ) ) ;
#9619=CARTESIAN_POINT ( 'NONE',  ( -221.2401356301573685, 146.6832912211113467, 9.651641063605101323 ) ) ;
#9622=AXIS2_PLACEMENT_3D ( 'NONE', #5393, #6816, #13826 ) ;
#9644=CARTESIAN_POINT ( 'NONE',  ( -225.4895753176805044, 143.2392427187964188, 4.987127499475484171 ) ) ;
#9650=EDGE_CURVE ( 'NONE', #1731, #14876, #304, .T. ) ;
#9666=CARTESIAN_POINT ( 'NONE',  ( -182.2196890910978482, 130.3369809632412739, -4.640918829492416187 ) ) ;
#9682=CARTESIAN_POINT ( 'NONE',  ( -217.9748787080196450, 139.5740753954225966, -0.4555467707853197989 ) ) ;
#9685=CARTESIAN_POINT ( 'NONE',  ( -192.4722482905459344, 130.7344553107722902, 9.577123744044227394 ) ) ;
#9696=EDGE_CURVE ( 'NONE', #3064, #14554, #3564, .T. ) ;
#9697=CARTESIAN_POINT ( 'NONE',  ( -223.3922821272916508, 142.4404936614456574, -0.2381634666249608234 ) ) ;
#9699=CARTESIAN_POINT ( 'NONE',  ( -223.5483852270401712, 142.1543297243506458, 4.029429640195547613 ) ) ;
#9702=CARTESIAN_POINT ( 'NONE',  ( -201.8658614229783268, 146.6084512934502584, 2.500000000000000000 ) ) ;
#9719=CARTESIAN_POINT ( 'NONE',  ( -224.5811800873043182, 144.8667753680073531, 1.831365460742872209 ) ) ;
#9723=CARTESIAN_POINT ( 'NONE',  ( -224.5735671299499927, 144.8804151761403034, 3.241364612890711427 ) ) ;
#9744=CARTESIAN_POINT ( 'NONE',  ( -187.0868153883506011, 133.8486679469899343, -4.640918829492425957 ) ) ;
#9758=CARTESIAN_POINT ( 'NONE',  ( -223.1255854116407420, 142.9625047383971719, -1.483432749446032206 ) ) ;
#9759=CARTESIAN_POINT ( 'NONE',  ( -224.7459018048070050, 144.5716505541534218, -3.023257939496649449 ) ) ;
#9762=CARTESIAN_POINT ( 'NONE',  ( -188.3680287392151627, 131.4989828868489781, 10.16010209732750269 ) ) ;
#9774=CARTESIAN_POINT ( 'NONE',  ( -177.3557003870508595, 132.9282874014947140, 2.500000000000000000 ) ) ;
#9787=CARTESIAN_POINT ( 'NONE',  ( -179.9311234670130943, 134.3555102485248369, 3.478855109513426580 ) ) ;
#9794=DIRECTION ( 'NONE',  ( -0.8731965799097684000, 0.4873681696970817989, 0.000000000000000000 ) ) ;
#9795=ORIENTED_EDGE ( 'NONE', *, *, #9048, .T. ) ;
#9796=CARTESIAN_POINT ( 'NONE',  ( -220.7954037378262058, 147.5269295839602535, 9.866320462745882480 ) ) ;
#9824=CARTESIAN_POINT ( 'NONE',  ( -208.4264987254875052, 144.6230976266233483, -4.640918829492436615 ) ) ;
#9840=CARTESIAN_POINT ( 'NONE',  ( -217.3067432674630197, 153.8362354792185158, -1.714361214038438552 ) ) ;
#9843=CARTESIAN_POINT ( 'NONE',  ( -179.8633755235878198, 122.3938961877832696, -4.689260562946571120 ) ) ;
#9847=CARTESIAN_POINT ( 'NONE',  ( -172.0064303153328638, 119.3480080297071595, 9.396848320176498959 ) ) ;
#9860=CARTESIAN_POINT ( 'NONE',  ( -207.1387806695930749, 146.9236570583465209, 7.919662025281895446 ) ) ;
#9864=ORIENTED_EDGE ( 'NONE', *, *, #2684, .T. ) ;
#9880=CARTESIAN_POINT ( 'NONE',  ( -221.8818932461130942, 149.7029714605600930, 7.941079238973655308 ) ) ;
#9882=CARTESIAN_POINT ( 'NONE',  ( -223.5913358527620005, 146.6402366934796078, 9.270357946057281140 ) ) ;
#9884=CARTESIAN_POINT ( 'NONE',  ( -173.5206377105050990, 117.3432113310319380, -2.605937114841728075 ) ) ;
#9903=CARTESIAN_POINT ( 'NONE',  ( -201.8658614229783268, 146.6084512934502584, 2.500000000000000000 ) ) ;
#9916=CARTESIAN_POINT ( 'NONE',  ( -223.0109838976775620, 143.1868724232609225, -1.877048790282907831 ) ) ;
#9917=APPLICATION_CONTEXT ( 'automotive_design' ) ;
#9918=CARTESIAN_POINT ( 'NONE',  ( -218.2851610432379346, 147.7600012847656217, -5.230826428279595319 ) ) ;
#9921=CARTESIAN_POINT ( 'NONE',  ( -222.1166800156826184, 149.2823141075699880, 10.12588066961105504 ) ) ;
#9931=CARTESIAN_POINT ( 'NONE',  ( -224.5272311401201648, 144.9634333754441400, 1.130582765288308034 ) ) ;
#9936=CARTESIAN_POINT ( 'NONE',  ( -199.6024142766798946, 142.8729305612646385, 7.919662025281897222 ) ) ;
#9949=CARTESIAN_POINT ( 'NONE',  ( -169.9361637590235716, 128.7768979049109532, 3.478855110294483133 ) ) ;
#9961=CARTESIAN_POINT ( 'NONE',  ( -220.9030130636566298, 151.4567889657070339, 9.535387874750053783 ) ) ;
#9963=CARTESIAN_POINT ( 'NONE',  ( -167.8857020579134200, 127.4390830883378953, 0.6628302033481980882 ) ) ;
#9983=CARTESIAN_POINT ( 'NONE',  ( -198.5677679834141713, 144.7676449960911498, 2.500000000000000000 ) ) ;
#9997=CARTESIAN_POINT ( 'NONE',  ( -221.8246199127426053, 145.4969522655044329, -4.202312765555400453 ) ) ;
#9998=CARTESIAN_POINT ( 'NONE',  ( -184.7739606708014719, 119.6463200498024548, -0.4555467707853387282 ) ) ;
#10001=CARTESIAN_POINT ( 'NONE',  ( -181.0973828845548610, 120.1829782941312743, 7.859965607560862821 ) ) ;
#10025=CARTESIAN_POINT ( 'NONE',  ( -219.4693564981101588, 154.0254097489945764, 1.294062626199961930 ) ) ;
#10026=CARTESIAN_POINT ( 'NONE',  ( -172.3625742532922800, 130.1311808564658747, 3.478855110039204224 ) ) ;
#10032=CARTESIAN_POINT ( 'NONE',  ( -221.8843987189232507, 149.6984825127276224, 7.941366815851232275 ) ) ;
#10034=CARTESIAN_POINT ( 'NONE',  ( -170.8583098116105248, 122.1131896768847298, -5.150070920892065196 ) ) ;
#10068=CARTESIAN_POINT ( 'NONE',  ( -170.7063108826370694, 121.6823135672476752, -5.361935827173478941 ) ) ;
#10071=CARTESIAN_POINT ( 'NONE',  ( -182.0950013669840359, 118.3955881831737997, 1.446957622915671537 ) ) ;
#10085=CARTESIAN_POINT ( 'NONE',  ( -167.5097532647548633, 127.4226149533560175, 3.478855110549762042 ) ) ;
#10100=CARTESIAN_POINT ( 'NONE',  ( -217.1902381962481172, 154.0393758339013743, -1.351620443338561017 ) ) ;
#10110=CARTESIAN_POINT ( 'NONE',  ( -219.9563263261640316, 153.1529268606066125, 8.541693648944034933 ) ) ;
#10112=CARTESIAN_POINT ( 'NONE',  ( -171.0834245745559485, 121.7098612420110442, -5.167027133578317333 ) ) ;
#10134=CARTESIAN_POINT ( 'NONE',  ( -167.5053995445195767, 127.4304153265770907, 2.500000001036336350 ) ) ;
#10148=CARTESIAN_POINT ( 'NONE',  ( -192.3464331062453709, 140.8629472311621100, -0.4547266291960749829 ) ) ;
#10149=CARTESIAN_POINT ( 'NONE',  ( -223.5918188539070002, 142.0538562971642307, 1.612306317632525854 ) ) ;
#10151=CARTESIAN_POINT ( 'NONE',  ( -187.5349220100912930, 120.9938564418671518, 1.515400478619096658 ) ) ;
#10152=COLOUR_RGB ( '', 0.31764706, 0.68627451, 0.89019608) ;
#10163=CARTESIAN_POINT ( 'NONE',  ( -212.2525635541804547, 150.1126023820536375, 7.919662025281898998 ) ) ;
#10176=CARTESIAN_POINT ( 'NONE',  ( -216.8935220752126440, 154.5526377852563940, -0.02875724444948107861 ) ) ;
#10183=CARTESIAN_POINT ( 'NONE',  ( -220.4428784760894473, 152.2811923082724661, -1.958540667262526958 ) ) ;
#10185=ADVANCED_BREP_SHAPE_REPRESENTATION ( '', ( #10760, #12337 ), #4745 ) ;
#10187=CARTESIAN_POINT ( 'NONE',  ( -217.6921401408168322, 153.1680562725702828, 7.596881196942645964 ) ) ;
#10189=CARTESIAN_POINT ( 'NONE',  ( -171.1959741278963349, 121.5082110499024139, -5.161946524584423379 ) ) ;
#10204=EDGE_CURVE ( 'NONE', #13381, #3064, #6552, .T. ) ;
#10224=CARTESIAN_POINT ( 'NONE',  ( -207.1016862382755335, 146.9901175548950505, -2.963320117457100888 ) ) ;
#10227=CARTESIAN_POINT ( 'NONE',  ( -187.3366327499677197, 121.3409432500951937, 5.434137442415932107 ) ) ;
#10240=CARTESIAN_POINT ( 'NONE',  ( -198.4250122012724660, 129.4766065029076003, 7.918248976830634334 ) ) ;
#10250=CARTESIAN_POINT ( 'NONE',  ( -170.8822437509192582, 122.0703082676180884, 9.852955625550796626 ) ) ;
#10251=CARTESIAN_POINT ( 'NONE',  ( -218.1232943690431512, 152.3955998793410913, -3.540502677712229929 ) ) ;
#10260=CARTESIAN_POINT ( 'NONE',  ( -222.3080144202391466, 148.9395084873720521, -3.019567288535963900 ) ) ;
#10262=CARTESIAN_POINT ( 'NONE',  ( -217.8617492717439461, 152.8708317265722201, 7.945910111307878054 ) ) ;
#10279=ORIENTED_EDGE ( 'NONE', *, *, #859, .F. ) ;
#10301=CARTESIAN_POINT ( 'NONE',  ( -201.8614823352862970, 146.6162971164513635, 1.515441477536285220 ) ) ;
#10304=CARTESIAN_POINT ( 'NONE',  ( -214.8265656857867327, 135.2606554265309740, 3.478895870929493483 ) ) ;
#10312=CARTESIAN_POINT ( 'NONE',  ( -224.2094369203935003, 145.5328116053612746, 8.507951946043531777 ) ) ;
#10317=CARTESIAN_POINT ( 'NONE',  ( -214.7423002846986151, 145.5292334337732711, 10.16010209732751335 ) ) ;
#10330=CARTESIAN_POINT ( 'NONE',  ( -169.0248613439241012, 125.3981004096062435, 8.301827530276908007 ) ) ;
#10331=CARTESIAN_POINT ( 'NONE',  ( -219.6200563870737597, 153.7554072420239493, 0.2735799754665275696 ) ) ;
#10357=CARTESIAN_POINT ( 'NONE',  ( -223.6213244275821808, 142.0005027430226221, 2.566813877387965626 ) ) ;
#10377=CARTESIAN_POINT ( 'NONE',  ( -215.0356418556126812, 153.5741063705486908, -0.4547266291960771478 ) ) ;
#10380=CARTESIAN_POINT ( 'NONE',  ( -220.7908126485560274, 143.2766720833714089, -2.964974570226855288 ) ) ;
#10395=CARTESIAN_POINT ( 'NONE',  ( -195.8085210632896178, 134.3768662836672547, 10.16010209732750269 ) ) ;
#10406=CARTESIAN_POINT ( 'NONE',  ( -172.6089438593484147, 118.9766539771727452, 8.890414347921929306 ) ) ;
#10407=CARTESIAN_POINT ( 'NONE',  ( -223.5023877967964268, 146.7996010982761845, -2.058674291180297100 ) ) ;
#10416=CARTESIAN_POINT ( 'NONE',  ( -224.1052059537137495, 145.7195577436698954, -0.7975646616046745407 ) ) ;
#10440=CYLINDRICAL_SURFACE ( 'NONE', #14598, 4.499999999999950262 ) ;
#10458=CARTESIAN_POINT ( 'NONE',  ( -198.5633888957220563, 144.7754908190922549, 1.515441477536285442 ) ) ;
#10461=CARTESIAN_POINT ( 'NONE',  ( -205.7712766299887335, 131.5939592662764994, -0.4555467707853333992 ) ) ;
#10475=CARTESIAN_POINT ( 'NONE',  ( -197.2254974982137128, 131.7248478061943615, 9.577123744044225617 ) ) ;
#10485=CARTESIAN_POINT ( 'NONE',  ( -170.6576934677675581, 122.4726253483332812, 9.815104126961024633 ) ) ;
#10486=CARTESIAN_POINT ( 'NONE',  ( -222.7865639444310943, 148.0821118951906215, -4.926004749479361955 ) ) ;
#10528=CARTESIAN_POINT ( 'NONE',  ( -207.1238489746795608, 137.1336079999123854, -4.642206099735007641 ) ) ;
#10545=CARTESIAN_POINT ( 'NONE',  ( -194.3889542450793613, 137.0335258394182745, 9.578254705571838556 ) ) ;
#10558=CARTESIAN_POINT ( 'NONE',  ( -168.2037493089125348, 126.8692515131764367, 6.097242495366466564 ) ) ;
#10559=CARTESIAN_POINT ( 'NONE',  ( -223.3602385083506761, 147.0542838622007480, -2.257390889150600266 ) ) ;
#10560=CARTESIAN_POINT ( 'NONE',  ( -216.7960616128559650, 154.7191080884769860, 4.212816267783609625 ) ) ;
#10573=CARTESIAN_POINT ( 'NONE',  ( -219.4360840196857509, 154.0850226169902442, 3.058976617611885107 ) ) ;
#10608=ORIENTED_EDGE ( 'NONE', *, *, #9696, .F. ) ;
#10616=CARTESIAN_POINT ( 'NONE',  ( -218.2851610432379346, 147.7600012847656217, -5.230826428279595319 ) ) ;
#10629=CARTESIAN_POINT ( 'NONE',  ( -221.7331157600676192, 141.5908957077777188, 1.515400478619091551 ) ) ;
#10641=CARTESIAN_POINT ( 'NONE',  ( -222.9903997373972402, 143.2271625030612086, -1.944083899231426882 ) ) ;
#10643=CARTESIAN_POINT ( 'NONE',  ( -221.5485735812534358, 146.0927223962365531, 9.417135290729820696 ) ) ;
#10649=CARTESIAN_POINT ( 'NONE',  ( -169.9318100387881714, 128.7846982781319412, 2.500000000781056997 ) ) ;
#10654=( NAMED_UNIT ( * ) SI_UNIT ( $, .STERADIAN. ) SOLID_ANGLE_UNIT ( ) );
#10658=( GEOMETRIC_REPRESENTATION_CONTEXT ( 3 ) GLOBAL_UNCERTAINTY_ASSIGNED_CONTEXT ( ( #12732 ) ) GLOBAL_UNIT_ASSIGNED_CONTEXT ( ( #13281, #2330, #6924 ) ) REPRESENTATION_CONTEXT ( 'NONE', 'WORKASPACE' ) );
#10660=CARTESIAN_POINT ( 'NONE',  ( -192.1704923257120754, 141.1970532186197431, 2.500000000000000000 ) ) ;
#10693=CARTESIAN_POINT ( 'NONE',  ( -213.7219974575431252, 137.2233070386400584, -2.964974570226852180 ) ) ;
#10707=CARTESIAN_POINT ( 'NONE',  ( -221.5581585947747101, 141.9038310245542505, 5.434137442415940988 ) ) ;
#10719=CARTESIAN_POINT ( 'NONE',  ( -221.3544506110429495, 150.6479677358152856, -4.921649773945601325 ) ) ;
#10720=CARTESIAN_POINT ( 'NONE',  ( -223.6012825982128902, 142.0449791388664664, 3.334463815293894573 ) ) ;
#10734=CARTESIAN_POINT ( 'NONE',  ( -187.9132138465967898, 138.8208849330412988, 2.500000000000000000 ) ) ;
#10738=CARTESIAN_POINT ( 'NONE',  ( -206.0222741447286126, 148.9180917377961464, 3.478855109513426580 ) ) ;
#10749=CARTESIAN_POINT ( 'NONE',  ( -224.3063355247866468, 145.3592025451120833, 8.356870423832322814 ) ) ;
#10759=CARTESIAN_POINT ( 'NONE',  ( -220.3531759299249302, 148.3382346779569616, 2.431557144026069928 ) ) ;
#10760=MANIFOLD_SOLID_BREP ( 'Cut-Extrude9', #6882 ) ;
#10766=CARTESIAN_POINT ( 'NONE',  ( -192.1704923257120754, 141.1970532186197431, 2.500000000000000000 ) ) ;
#10770=CARTESIAN_POINT ( 'NONE',  ( -171.9495551447802200, 125.1641050887067053, -4.702677209512893697 ) ) ;
#10786=CARTESIAN_POINT ( 'NONE',  ( -199.2256335332332640, 127.9713659812714042, 5.434137442415931218 ) ) ;
#10789=CARTESIAN_POINT ( 'NONE',  ( -198.4250122012724660, 129.4766065029076003, 7.918248976830634334 ) ) ;
#10821=CARTESIAN_POINT ( 'NONE',  ( -218.4444600228138711, 155.8616726660956715, 2.500000000270498735 ) ) ;
#10832=CARTESIAN_POINT ( 'NONE',  ( -224.5838421180054070, 144.8620059220666008, 7.877574876664438008 ) ) ;
#10850=CARTESIAN_POINT ( 'NONE',  ( -222.8347869274849415, 143.8920390286132829, 1.831365460742872209 ) ) ;
#10855=CARTESIAN_POINT ( 'NONE',  ( -211.4625087271040513, 151.5689812133889234, -0.4547266291960755935 ) ) ;
#10871=CARTESIAN_POINT ( 'NONE',  ( -209.2398179475638926, 133.3202902034983595, 5.434137442415948094 ) ) ;
#10874=CARTESIAN_POINT ( 'NONE',  ( -189.6066827460468858, 129.2255495722319836, 9.577123744044220288 ) ) ;
#10879=CARTESIAN_POINT ( 'NONE',  ( -194.4336556300434893, 127.2574632897803326, 2.431555724346868175 ) ) ;
#10884=CARTESIAN_POINT ( 'NONE',  ( -225.6712625649270478, 142.9137214952622514, 1.583163137451349511 ) ) ;
#10885=CARTESIAN_POINT ( 'NONE',  ( -222.4620031969695049, 144.3197956335804122, 8.205567776478527975 ) ) ;
#10911=STYLED_ITEM ( 'NONE', ( #11809 ), #10760 ) ;
#10912=CARTESIAN_POINT ( 'NONE',  ( -223.0117914826104766, 143.2331855431448560, 6.837811219071827651 ) ) ;
#10932=CARTESIAN_POINT ( 'NONE',  ( -202.0520865685784884, 146.2723300204251018, -0.4547266291960743168 ) ) ;
#10948=CARTESIAN_POINT ( 'NONE',  ( -217.9771163551940276, 139.5700662992579737, 5.434137442415948982 ) ) ;
#10952=CARTESIAN_POINT ( 'NONE',  ( -198.9139648670198994, 132.3922632189928095, 9.577123744044227394 ) ) ;
#10979=CARTESIAN_POINT ( 'NONE',  ( -206.8718859864436581, 149.4025266312245037, 2.500000000000000000 ) ) ;
#10986=CARTESIAN_POINT ( 'NONE',  ( -223.0208697908820739, 147.6623161915171636, 9.682315826541753268 ) ) ;
#11006=CARTESIAN_POINT ( 'NONE',  ( -177.5434268683390826, 132.5922366007948199, -0.4547266291960713747 ) ) ;
#11019=CARTESIAN_POINT ( 'NONE',  ( -177.2366359034146512, 121.3924996022181375, -4.733667549831950261 ) ) ;
#11023=CARTESIAN_POINT ( 'NONE',  ( -223.5464781713420734, 146.7206062712571111, 9.530069280832668355 ) ) ;
#11048=CARTESIAN_POINT ( 'NONE',  ( -187.9132138465967898, 138.8208849330412988, 2.500000000000000000 ) ) ;
#11058=CARTESIAN_POINT ( 'NONE',  ( -223.5526519068884852, 142.1455622009127637, 3.981868244017999992 ) ) ;
#11061=CARTESIAN_POINT ( 'NONE',  ( -173.0510230909240192, 118.1845996390716351, -3.619230586480127076 ) ) ;
#11099=CARTESIAN_POINT ( 'NONE',  ( -213.3556830655219585, 148.0789703896194567, -4.640918829492433950 ) ) ;
#11103=CARTESIAN_POINT ( 'NONE',  ( -174.5069932933876942, 126.2863744793834826, 9.536681319450917016 ) ) ;
#11116=CARTESIAN_POINT ( 'NONE',  ( -198.7725242955204692, 144.3921638819772113, 5.434754235172606585 ) ) ;
#11132=CARTESIAN_POINT ( 'NONE',  ( -178.4232521731099439, 131.0169814278324907, 7.919662025281895446 ) ) ;
#11138=CARTESIAN_POINT ( 'NONE',  ( -224.2481407916400542, 145.4634675445406913, 5.252818170846536461 ) ) ;
#11140=CARTESIAN_POINT ( 'NONE',  ( -220.4524996695633092, 148.1714595847825819, 9.941101666187114105 ) ) ;
#11162=CARTESIAN_POINT ( 'NONE',  ( -211.2987210398670186, 151.8733316563206586, 2.500000000000000000 ) ) ;
#11177=CARTESIAN_POINT ( 'NONE',  ( -223.3976496709624939, 142.4299982425674216, -0.2056757461415917587 ) ) ;
#11178=CARTESIAN_POINT ( 'NONE',  ( -200.9686762702122849, 128.5620043109015853, -0.4555467707853345649 ) ) ;
#11181=CARTESIAN_POINT ( 'NONE',  ( -175.7482920159357604, 118.3486081613139334, 7.749957389927518925 ) ) ;
#11192=CARTESIAN_POINT ( 'NONE',  ( -206.8762397066792005, 149.3947262580036863, 3.478855109513426580 ) ) ;
#11206=CARTESIAN_POINT ( 'NONE',  ( -219.7707515677084302, 153.4854131707639340, -0.3598758021188548373 ) ) ;
#11207=CARTESIAN_POINT ( 'NONE',  ( -219.4661802592007689, 154.0311004795854046, 7.909502539118774322 ) ) ;
#11214=CARTESIAN_POINT ( 'NONE',  ( -223.8340338030139094, 146.2054052184961961, 6.383663356545733691 ) ) ;
#11215=ORIENTED_EDGE ( 'NONE', *, *, #4283, .F. ) ;
#11216=CARTESIAN_POINT ( 'NONE',  ( -221.1271579233365969, 151.0551982647748446, 7.614349089095027168 ) ) ;
#11218=CARTESIAN_POINT ( 'NONE',  ( -167.8641735700121558, 127.4776547538155853, 0.8902203665584077497 ) ) ;
#11230=EDGE_LOOP ( 'NONE', ( #11710, #6697, #14732, #12100 ) ) ;
#11249=CARTESIAN_POINT ( 'NONE',  ( -219.9272211304954681, 149.1032166049582486, -5.025525059679186057 ) ) ;
#11250=CARTESIAN_POINT ( 'NONE',  ( -173.7777028115792177, 116.1670890754947152, -0.7095712321138001322 ) ) ;
#11254=CARTESIAN_POINT ( 'NONE',  ( -187.5349220100912930, 120.9938564418671518, 3.478895870929501921 ) ) ;
#11268=CARTESIAN_POINT ( 'NONE',  ( -177.3600541072865155, 132.9204870282739819, 3.478855109513427468 ) ) ;
#11278=CARTESIAN_POINT ( 'NONE',  ( -217.5316743144719567, 153.4425273680139696, -2.341497464274004070 ) ) ;
#11283=CARTESIAN_POINT ( 'NONE',  ( -221.0392844523545364, 151.2126373818472871, -2.672071522959135415 ) ) ;
#11285=CARTESIAN_POINT ( 'NONE',  ( -220.1509919453162638, 152.8041528465324461, 8.810372448773614806 ) ) ;
#11287=CARTESIAN_POINT ( 'NONE',  ( -169.5742008144607098, 124.4138725163886505, -4.326550720942743844 ) ) ;
#11313=CARTESIAN_POINT ( 'NONE',  ( -223.6145774380523505, 142.0129443944823606, 2.393984899497048513 ) ) ;
#11324=CARTESIAN_POINT ( 'NONE',  ( -191.1563096742665380, 133.0698578461479826, -5.230826428279597984 ) ) ;
#11327=CARTESIAN_POINT ( 'NONE',  ( -179.3772030532177837, 117.5545944912402661, 1.382365641875445528 ) ) ;
#11355=CARTESIAN_POINT ( 'NONE',  ( -219.5587625787842114, 153.8652247210798123, 0.6104961448661524459 ) ) ;
#11370=CARTESIAN_POINT ( 'NONE',  ( -216.9389196770082151, 154.4740194435295564, 5.145036412574403251 ) ) ;
#11372=CARTESIAN_POINT ( 'NONE',  ( -172.3934359946532311, 119.3627701458021875, -4.525325099609154300 ) ) ;
#11390=CARTESIAN_POINT ( 'NONE',  ( -177.3557003870508595, 132.9282874014947140, 2.500000000000000000 ) ) ;
#11404=CARTESIAN_POINT ( 'NONE',  ( -173.2995934586704152, 128.4510609142004114, -2.983067475588502937 ) ) ;
#11408=CARTESIAN_POINT ( 'NONE',  ( -191.4964613557999655, 125.7493975051623352, 3.478895870929489043 ) ) ;
#11412=AXIS2_PLACEMENT_3D ( 'NONE', #3697, #14578, #8526 ) ;
#11420=CARTESIAN_POINT ( 'NONE',  ( -183.7478807014743722, 127.6480629723144347, 10.16010209732750624 ) ) ;
#11442=CARTESIAN_POINT ( 'NONE',  ( -221.3648744334925027, 150.6292918216330179, -2.896295222704587946 ) ) ;
#11445=CARTESIAN_POINT ( 'NONE',  ( -220.2190305748135586, 148.6074564430024054, 9.948829861901575811 ) ) ;
#11487=CARTESIAN_POINT ( 'NONE',  ( -194.7245433579248868, 140.1837011942588447, -2.963320117457102665 ) ) ;
#11490=CARTESIAN_POINT ( 'NONE',  ( -217.9771163551940276, 139.5700662992579737, 5.434137442415948982 ) ) ;
#11504=CARTESIAN_POINT ( 'NONE',  ( -189.9062345257129323, 135.2872556402745374, 9.578254705571842109 ) ) ;
#11514=CARTESIAN_POINT ( 'NONE',  ( -174.0411197980623399, 116.4106859692672629, 5.128256677369954275 ) ) ;
#11515=CARTESIAN_POINT ( 'NONE',  ( -220.8828325425079981, 151.4929455371446920, -2.526440128526473039 ) ) ;
#11522=CARTESIAN_POINT ( 'NONE',  ( -220.5827524466467082, 152.0305861335090185, -2.167411312480779007 ) ) ;
#11538=DIRECTION ( 'NONE',  ( 0.4873681696970831312, 0.8731965799097676229, 0.000000000000000000 ) ) ;
#11553=AXIS2_PLACEMENT_3D ( 'NONE', #7054, #5931, #3567 ) ;
#11559=CARTESIAN_POINT ( 'NONE',  ( -180.9555975561403613, 132.5588568579215973, -2.963320117457099112 ) ) ;
#11562=CARTESIAN_POINT ( 'NONE',  ( -197.4248861630254055, 135.1594620591177431, -5.230826428279599760 ) ) ;
#11575=CARTESIAN_POINT ( 'NONE',  ( -213.3956520262682091, 148.0073597223720583, 9.578254705571842109 ) ) ;
#11590=CARTESIAN_POINT ( 'NONE',  ( -169.8918728808606886, 123.8447131433307931, 9.392450650342059504 ) ) ;
#11591=CARTESIAN_POINT ( 'NONE',  ( -222.0684630521171528, 149.3687023665398499, -5.084110969117699774 ) ) ;
#11610=CARTESIAN_POINT ( 'NONE',  ( -206.0179204244930702, 148.9258921110169638, 2.500000000000000000 ) ) ;
#11643=CARTESIAN_POINT ( 'NONE',  ( -215.7895908902557380, 152.2252679817794956, -2.963320117457100444 ) ) ;
#11646=CARTESIAN_POINT ( 'NONE',  ( -220.6443225159919734, 151.9202736894074803, -4.662307221713795968 ) ) ;
#11663=CARTESIAN_POINT ( 'NONE',  ( -171.9895241055258168, 125.0924944214600885, 9.516496325551347724 ) ) ;
#11674=CARTESIAN_POINT ( 'NONE',  ( -170.3246542751710422, 123.0693173402045204, 9.678964735678034614 ) ) ;
#11675=CARTESIAN_POINT ( 'NONE',  ( -221.6215556288433675, 150.1694071680115883, -2.996691548334699196 ) ) ;
#11710=ORIENTED_EDGE ( 'NONE', *, *, #2684, .F. ) ;
#11720=CARTESIAN_POINT ( 'NONE',  ( -206.0179204244930702, 148.9258921110169638, 2.500000000000000000 ) ) ;
#11723=CARTESIAN_POINT ( 'NONE',  ( -224.7459018048070050, 144.5716505541534218, -3.023257939496649449 ) ) ;
#11738=CARTESIAN_POINT ( 'NONE',  ( -192.4722482905459344, 130.7344553107722902, 9.577123744044227394 ) ) ;
#11749=CARTESIAN_POINT ( 'NONE',  ( -167.7990583880505824, 127.5943188236592363, 2.500000001005440620 ) ) ;
#11750=CARTESIAN_POINT ( 'NONE',  ( -222.0498794291082163, 149.4019978443419348, -3.065875947492658238 ) ) ;
#11751=CARTESIAN_POINT ( 'NONE',  ( -223.6145774380523505, 142.0129443944823606, 2.393984899497048513 ) ) ;
#11795=CARTESIAN_POINT ( 'NONE',  ( -209.2375803003894532, 133.3242992996629539, -0.4555467707853204096 ) ) ;
#11809=PRESENTATION_STYLE_ASSIGNMENT (( #11887 ) ) ;
#11813=CARTESIAN_POINT ( 'NONE',  ( -221.5559209476002991, 141.9078401207188449, -0.4555467707853290138 ) ) ;
#11826=CARTESIAN_POINT ( 'NONE',  ( -221.7378436215748820, 145.6645920127244835, -4.300707049757050093 ) ) ;
#11832=CARTESIAN_POINT ( 'NONE',  ( -172.3582205330567945, 130.1389812296867774, 2.500000000525777644 ) ) ;
#11838=CARTESIAN_POINT ( 'NONE',  ( -216.6986482686336331, 154.8858946472299465, 2.630718524060158714 ) ) ;
#11842=CARTESIAN_POINT ( 'NONE',  ( -216.6980668629938123, 154.8869363267023687, 2.500000000158653091 ) ) ;
#11875=CARTESIAN_POINT ( 'NONE',  ( -201.8658614229783268, 146.6084512934502584, 2.500000000000000000 ) ) ;
#11879=CARTESIAN_POINT ( 'NONE',  ( -182.6467173238959560, 123.4549944991208292, -4.642206099735001423 ) ) ;
#11887=SURFACE_STYLE_USAGE ( .BOTH. , #7239 ) ;
#11891=CARTESIAN_POINT ( 'NONE',  ( -173.9416064256852508, 115.8726071073731987, 1.253181679794994174 ) ) ;
#11903=CARTESIAN_POINT ( 'NONE',  ( -222.8935454358862387, 147.8904377599758391, -2.724937377524569104 ) ) ;
#11904=CARTESIAN_POINT ( 'NONE',  ( -223.4402560244223821, 142.3745948123178664, 4.936224999423321158 ) ) ;
#11932=CARTESIAN_POINT ( 'NONE',  ( -225.4016773603011927, 143.3967257069427887, 5.447776948886904336 ) ) ;
#11941=DIRECTION ( 'NONE',  ( 0.8731965799097684000, -0.4873681696970819655, 0.000000000000000000 ) ) ;
#11951=CARTESIAN_POINT ( 'NONE',  ( -185.2055264765504887, 137.3096093875189467, 2.500000000000000000 ) ) ;
#11955=CARTESIAN_POINT ( 'NONE',  ( -185.2011473888584874, 137.3174552105199666, 1.515441477536283887 ) ) ;
#11962=EDGE_CURVE ( 'NONE', #14876, #13381, #4516, .T. ) ;
#11971=CARTESIAN_POINT ( 'NONE',  ( -191.3393351389284192, 126.0399454915928317, 5.434137442415923225 ) ) ;
#11974=CARTESIAN_POINT ( 'NONE',  ( -214.7423002846986151, 145.5292334337732711, 10.16010209732751335 ) ) ;
#11978=CARTESIAN_POINT ( 'NONE',  ( -182.0948474510348092, 118.3958639477576043, 2.363114587883560436 ) ) ;
#11986=CARTESIAN_POINT ( 'NONE',  ( -217.1827905065508446, 154.0535767968314644, 6.164366753867413173 ) ) ;
#11989=CARTESIAN_POINT ( 'NONE',  ( -192.1704923257120754, 141.1970532186197431, 2.500000000000000000 ) ) ;
#12000=CARTESIAN_POINT ( 'NONE',  ( -214.8715905313398480, 153.8675021612092451, 2.500000000000000000 ) ) ;
#12009=CARTESIAN_POINT ( 'NONE',  ( -222.6685243335228677, 148.2935983871826977, 9.839440528619144644 ) ) ;
#12025=CARTESIAN_POINT ( 'NONE',  ( -219.4290858278833980, 154.0975609761335932, -2.973479603620232226 ) ) ;
#12039=CARTESIAN_POINT ( 'NONE',  ( -181.0973828845548610, 120.1829782941312743, 7.859965607560862821 ) ) ;
#12042=CARTESIAN_POINT ( 'NONE',  ( -210.8662606591548752, 142.3010704693858486, 10.16010209732750624 ) ) ;
#12053=CARTESIAN_POINT ( 'NONE',  ( -223.0788147039891953, 143.0998217501368401, 6.615244852604288184 ) ) ;
#12079=CARTESIAN_POINT ( 'NONE',  ( -223.1412712182228972, 147.4465981345315981, 7.416791562717193642 ) ) ;
#12100=ORIENTED_EDGE ( 'NONE', *, *, #1378, .F. ) ;
#12101=CARTESIAN_POINT ( 'NONE',  ( -173.2995934586704152, 128.4510609142004114, -2.983067475588502937 ) ) ;
#12116=CARTESIAN_POINT ( 'NONE',  ( -173.0737465816261818, 117.4314230949052558, 7.694953281110847421 ) ) ;
#12121=CARTESIAN_POINT ( 'NONE',  ( -170.7405378081422214, 121.6209906574826931, 10.02899269843361374 ) ) ;
#12127=CARTESIAN_POINT ( 'NONE',  ( -174.2824251065520968, 115.9783496305641535, 2.177446462082195389 ) ) ;
#12132=CARTESIAN_POINT ( 'NONE',  ( -225.4439234422023617, 143.3210352198185547, -0.3244446825575932891 ) ) ;
#12149=CARTESIAN_POINT ( 'NONE',  ( -192.1748460459477030, 141.1892528453990110, 3.478855109513427468 ) ) ;
#12157=CARTESIAN_POINT ( 'NONE',  ( -223.4491651843841282, 142.3567805253620691, 4.912650739265252753 ) ) ;
#12177=CARTESIAN_POINT ( 'NONE',  ( -185.3517468524019591, 137.0386009272039871, -0.4547266291960738172 ) ) ;
#12178=CARTESIAN_POINT ( 'NONE',  ( -223.6145774380523505, 142.0129443944823606, 2.393984899497048513 ) ) ;
#12189=CARTESIAN_POINT ( 'NONE',  ( -218.3491273834486890, 151.9915237902018248, -3.871359521417834237 ) ) ;
#12190=CARTESIAN_POINT ( 'NONE',  ( -191.3370974917540366, 126.0439545877573266, -0.4555467707853441128 ) ) ;
#12193=CARTESIAN_POINT ( 'NONE',  ( -178.4568510201948186, 124.9139056227158733, 10.12588066961104261 ) ) ;
#12229=CARTESIAN_POINT ( 'NONE',  ( -224.6033116245361043, 144.8271232449910713, 2.544233000457407634 ) ) ;
#12231=CARTESIAN_POINT ( 'NONE',  ( -224.9759671128498439, 144.1594524405806510, 6.941577500106505205 ) ) ;
#12233=CARTESIAN_POINT ( 'NONE',  ( -171.4210576570572471, 121.1049385752565541, -5.124804266949916531 ) ) ;
#12252=CARTESIAN_POINT ( 'NONE',  ( -211.2943419521749888, 151.8811774793218490, 1.515441477536285220 ) ) ;
#12264=CARTESIAN_POINT ( 'NONE',  ( -218.5464654778641034, 151.6367060758224454, -4.121322150339921109 ) ) ;
#12265=CARTESIAN_POINT ( 'NONE',  ( -216.9311889273521672, 150.1826874172201656, -4.640918829492440167 ) ) ;
#12269=CARTESIAN_POINT ( 'NONE',  ( -175.8847466161772957, 123.8162673009714752, 10.09358467921856573 ) ) ;
#12279=CARTESIAN_POINT ( 'NONE',  ( -185.3757041553864156, 136.9956776582455973, 5.434754235172603920 ) ) ;
#12295=CARTESIAN_POINT ( 'NONE',  ( -177.3600541072865155, 132.9204870282739819, 3.478855109513427468 ) ) ;
#12305=CARTESIAN_POINT ( 'NONE',  ( -216.7483548245723455, 154.8006932417845860, 3.755670596743044598 ) ) ;
#12330=CARTESIAN_POINT ( 'NONE',  ( -179.9267697467775520, 134.3633106217456543, 2.500000000000000000 ) ) ;
#12337=AXIS2_PLACEMENT_3D ( 'NONE', #4568, #8147, #5681 ) ;
#12344=CARTESIAN_POINT ( 'NONE',  ( -223.2729691302634194, 142.6739754659882919, -0.8558400769978052880 ) ) ;
#12346=CARTESIAN_POINT ( 'NONE',  ( -204.9433645127610646, 133.1096489332827275, -2.964974570226844186 ) ) ;
#12350=CARTESIAN_POINT ( 'NONE',  ( -194.4337897068680547, 127.2572260587109554, 1.515400478619095992 ) ) ;
#12378=CARTESIAN_POINT ( 'NONE',  ( -188.0905678060899220, 138.5068454852687125, 5.434754235172603920 ) ) ;
#12385=CARTESIAN_POINT ( 'NONE',  ( -171.4541674549778065, 121.0456171749203520, 2.431557144026069928 ) ) ;
#12387=CARTESIAN_POINT ( 'NONE',  ( -219.4906815929313950, 153.9872024941471693, 3.763993901578424062 ) ) ;
#12421=CARTESIAN_POINT ( 'NONE',  ( -216.9004380970166039, 154.5406409916104735, -0.03430832140138441455 ) ) ;
#12422=CARTESIAN_POINT ( 'NONE',  ( -209.9898587843626956, 141.8296236499265035, -5.230826428279598872 ) ) ;
#12425=CARTESIAN_POINT ( 'NONE',  ( -205.9652191273047777, 131.2378527988410326, 3.478895870929496148 ) ) ;
#12439=CARTESIAN_POINT ( 'NONE',  ( -177.5673841713239085, 132.5493133318365437, 5.434754235172600367 ) ) ;
#12454=CARTESIAN_POINT ( 'NONE',  ( -221.0392844523455267, 151.2126373818634306, -2.672071523003486160 ) ) ;
#12455=CARTESIAN_POINT ( 'NONE',  ( -192.3703904092303105, 140.8200239622036918, 5.434754235172604808 ) ) ;
#12462=CARTESIAN_POINT ( 'NONE',  ( -221.6258104990438937, 150.1617839001448260, 7.894136746929314441 ) ) ;
#12464=CARTESIAN_POINT ( 'NONE',  ( -168.0753201600388422, 127.0993524933591630, -0.6766640714057908790 ) ) ;
#12497=CARTESIAN_POINT ( 'NONE',  ( -223.5232045190763301, 146.7623046726374980, -4.689260562946596878 ) ) ;
#12500=CARTESIAN_POINT ( 'NONE',  ( -213.7863261933728154, 135.0464837791089963, 5.434137442415932995 ) ) ;
#12512=ORIENTED_EDGE ( 'NONE', *, *, #11962, .T. ) ;
#12514=CARTESIAN_POINT ( 'NONE',  ( -172.5511497006709192, 129.7930440361603246, 5.430596897033706405 ) ) ;
#12525=CARTESIAN_POINT ( 'NONE',  ( -218.4739499160498042, 155.8088368932420167, 1.364465161875672239 ) ) ;
#12526=ORIENTED_EDGE ( 'NONE', *, *, #13028, .F. ) ;
#12534=CARTESIAN_POINT ( 'NONE',  ( -219.9184004181287264, 153.2208770782757767, 5.686502709355995222 ) ) ;
#12535=EDGE_LOOP ( 'NONE', ( #12526, #13252, #7208, #3252, #8468 ) ) ;
#12570=CARTESIAN_POINT ( 'NONE',  ( -192.1661132380199604, 141.2048990416207630, 1.515441477536284332 ) ) ;
#12573=CARTESIAN_POINT ( 'NONE',  ( -173.9416064256852508, 115.8726071073731987, 3.216677072105399660 ) ) ;
#12592=CARTESIAN_POINT ( 'NONE',  ( -212.8994228580217509, 136.6308034654096559, 7.918248976830621011 ) ) ;
#12608=CARTESIAN_POINT ( 'NONE',  ( -220.0724991394466485, 152.9447850296163836, -1.223998976583901444 ) ) ;
#12620=CARTESIAN_POINT ( 'NONE',  ( -219.8231187948979652, 153.3915890629854744, 5.390158053389423110 ) ) ;
#12653=CARTESIAN_POINT ( 'NONE',  ( -180.1141531658810777, 134.0357633396332915, -0.4547266291960706530 ) ) ;
#12656=CARTESIAN_POINT ( 'NONE',  ( -176.6594047394515314, 116.7136007993067324, 3.281269053145625225 ) ) ;
#12663=CARTESIAN_POINT ( 'NONE',  ( -220.3531759299249302, 148.3382346779569616, 2.431557144026069928 ) ) ;
#12668=CARTESIAN_POINT ( 'NONE',  ( -203.7296541848517109, 135.3294987143146955, 9.577123744044227394 ) ) ;
#12681=CARTESIAN_POINT ( 'NONE',  ( -169.2966169123036480, 124.9112076504258368, 8.722866747349085514 ) ) ;
#12682=CARTESIAN_POINT ( 'NONE',  ( -219.8602732318529434, 153.3250210569181320, -0.6604898282866703552 ) ) ;
#12728=CARTESIAN_POINT ( 'NONE',  ( -168.3602667112202766, 125.8948777600411830, -3.002243219525047024 ) ) ;
#12731=CARTESIAN_POINT ( 'NONE',  ( -200.9686762702122849, 128.5620043109015853, -0.4555467707853345649 ) ) ;
#12732=UNCERTAINTY_MEASURE_WITH_UNIT (LENGTH_MEASURE( 1.000000000000000082E-05 ), #13281, 'distance_accuracy_value', 'NONE');
#12735=B_SPLINE_CURVE_WITH_KNOTS ( 'NONE', 3,
 ( #15507, #6136, #1073, #6062, #4706, #9527, #5233, #13382, #8587, #10879, #4872, #395, #13057, #11978, #8511, #8440, #12127 ),
 .UNSPECIFIED., .F., .F.,
 ( 4, 2, 2, 2, 2, 2, 3, 4 ),
 ( 0.04448509752560573377, 0.2455027589669699362, 0.3041813370740077405, 0.5308033955276699745, 0.6372805264318514018, 0.8233339832829627003, 0.9999999999999998890, 1.159754059773842050 ),
 .UNSPECIFIED. ) ;
#12747=CARTESIAN_POINT ( 'NONE',  ( -200.8348121886614024, 140.6195990399117477, 9.578254705571838556 ) ) ;
#12759=CARTESIAN_POINT ( 'NONE',  ( -169.5864954465999972, 124.3918447529796509, 9.093140960474290324 ) ) ;
#12768=CARTESIAN_POINT ( 'NONE',  ( -223.3602385079212524, 147.0542838629705500, -2.257390888005822216 ) ) ;
#12800=PRODUCT_DEFINITION_SHAPE ( 'NONE', 'NONE',  #6635 ) ;
#12806=CARTESIAN_POINT ( 'NONE',  ( -202.0520865685784884, 146.2723300204251018, -0.4547266291960743168 ) ) ;
#12809=CARTESIAN_POINT ( 'NONE',  ( -216.0630845075784805, 143.0974466248333954, -4.642206099735013858 ) ) ;
#12825=CARTESIAN_POINT ( 'NONE',  ( -181.1823003367078115, 126.0769834546670296, 10.16010209732750624 ) ) ;
#12837=CARTESIAN_POINT ( 'NONE',  ( -167.9557412913654844, 127.3135968073034974, 4.793417203503699930 ) ) ;
#12840=CARTESIAN_POINT ( 'NONE',  ( -220.6535933262513822, 147.7382320429851177, -5.005762723283130100 ) ) ;
#12890=CARTESIAN_POINT ( 'NONE',  ( -207.9521514620915639, 147.4834172152791325, -2.963320117457100888 ) ) ;
#12893=CARTESIAN_POINT ( 'NONE',  ( -181.9037801448002938, 118.7381910193847716, -0.5218507872395746761 ) ) ;
#12909=CARTESIAN_POINT ( 'NONE',  ( -197.4591130885309553, 135.0981391493542105, 10.16010209732750802 ) ) ;
#12911=DIRECTION ( 'NONE',  ( 0.8731965799097682890, -0.4873681696970819099, -0.000000000000000000 ) ) ;
#12921=CARTESIAN_POINT ( 'NONE',  ( -173.1348595683955978, 118.0343934295742656, 8.028916588137546384 ) ) ;
#12922=CARTESIAN_POINT ( 'NONE',  ( -221.1215437059437647, 151.0652570165180748, -4.807651471730975068 ) ) ;
#12923=CARTESIAN_POINT ( 'NONE',  ( -216.7478739536621504, 154.8015167611612810, 3.747099613486799097 ) ) ;
#12966=( BOUNDED_SURFACE ( )  B_SPLINE_SURFACE ( 3, 2, ( 
 ( #3476, #7046, #5854 ),
 ( #6738, #700, #3328 ),
 ( #10357, #9184, #15153 ),
 ( #14052, #8167, #8086 ),
 ( #867, #5699, #9723 ),
 ( #11058, #7362, #1176 ),
 ( #2612, #4737, #7130 ),
 ( #12157, #9644, #2449 ),
 ( #3559, #11932, #1409 ),
 ( #14440, #8314, #1335 ),
 ( #3636, #6008, #2376 ),
 ( #2295, #8469, #13097 ),
 ( #10912, #12231, #6244 ),
 ( #6094, #1105, #8616 ),
 ( #5924, #10832, #15534 ),
 ( #8398, #10749, #6174 ),
 ( #209, #10312, #68 ),
 ( #7209, #13251, #14593 ),
 ( #4907, #9561, #7282 ),
 ( #5057, #9882, #12079 ),
 ( #14672, #14363, #4823 ),
 ( #1258, #10986, #136 ),
 ( #14516, #13176, #3710 ),
 ( #8539, #12009, #13330 ),
 ( #9796, #2532, #4979 ),
 ( #3794, #13414, #7436 ),
 ( #11140, #4017, #13561 ),
 ( #11445, #2848, #8850 ),
 ( #3872, #1571, #10032 ),
 ( #369, #7672, #12462 ),
 ( #6408, #1806, #14819 ),
 ( #13641, #9961, #14902 ),
 ( #14977, #1651, #11216 ),
 ( #4097, #294, #5287 ),
 ( #6646, #611, #6488 ),
 ( #5134, #11285, #5210 ),
 ( #446, #10110, #13800 ),
 ( #10262, #14747, #3945 ),
 ( #10187, #3000, #8696 ),
 ( #8931, #5448, #2927 ),
 ( #2768, #4168, #12534 ),
 ( #13725, #7832, #12620 ),
 ( #13486, #7751, #1727 ),
 ( #2690, #8766, #6567 ),
 ( #11370, #7592, #529 ),
 ( #5366, #7509, #12387 ),
 ( #12305, #9006, #1490 ),
 ( #6328, #6792, #10573 ) ),
 .UNSPECIFIED., .F., .F., .T. ) 
 B_SPLINE_SURFACE_WITH_KNOTS ( ( 4, 2, 2, 2, 2, 2, 2, 2, 2, 2, 2, 2, 2, 2, 2, 2, 2, 2, 2, 2, 2, 2, 2, 4 ),
 ( 3, 3 ),
 ( 0.000000000000000000, 0.001056470869493305806, 0.001584706304239958709, 0.002112941738986611612, 0.003169412608479917418, 0.003697648043226570320, 0.004225883477973223223, 0.005282354347466529029, 0.005810589782213181932, 0.006338825216959834835, 0.007395296086453140641, 0.007923531521199792677, 0.008451766955946446447, 0.008980002390693100217, 0.009508237825439752253, 0.01056470869493305806, 0.01109294412967971183, 0.01162117956442636386, 0.01267765043391966967, 0.01373412130341297548, 0.01426235673815962751, 0.01479059217290628128, 0.01584706304239958535, 0.01690353391189289289 ),
 ( 0.000000000000000000, 1.000000000000000000 ),
 .UNSPECIFIED. ) 
 GEOMETRIC_REPRESENTATION_ITEM ( )  RATIONAL_B_SPLINE_SURFACE ( (
 ( 1.000000000000000000, 0.6642977373962596355, 1.000000000000000000),
 ( 1.000000000000000000, 0.6640838462638519735, 1.000000000000000000),
 ( 1.000000000000000000, 0.6642530361896505919, 1.000000000000000000),
 ( 1.000000000000000000, 0.6650420274440705937, 1.000000000000000000),
 ( 1.000000000000000000, 0.6653930490377342188, 1.000000000000000000),
 ( 1.000000000000000000, 0.6662696147822118053, 1.000000000000000000),
 ( 1.000000000000000000, 0.6667987513150220868, 1.000000000000000000),
 ( 1.000000000000000000, 0.6686259794347244600, 1.000000000000000000),
 ( 1.000000000000000000, 0.6701877536239834177, 1.000000000000000000),
 ( 1.000000000000000000, 0.6729075291465889119, 1.000000000000000000),
 ( 1.000000000000000000, 0.6738761219039702821, 1.000000000000000000),
 ( 1.000000000000000000, 0.6759369341149453758, 1.000000000000000000),
 ( 1.000000000000000000, 0.6770267051557863347, 1.000000000000000000),
 ( 1.000000000000000000, 0.6804085633467442662, 1.000000000000000000),
 ( 1.000000000000000000, 0.6828728915351610640, 1.000000000000000000),
 ( 1.000000000000000000, 0.6866515824972490023, 1.000000000000000000),
 ( 1.000000000000000000, 0.6879309149268769685, 1.000000000000000000),
 ( 1.000000000000000000, 0.6904804411488353333, 1.000000000000000000),
 ( 1.000000000000000000, 0.6917436029694029598, 1.000000000000000000),
 ( 1.000000000000000000, 0.6954928658986441192, 1.000000000000000000),
 ( 1.000000000000000000, 0.6979768248933013730, 1.000000000000000000),
 ( 1.000000000000000000, 0.7014000669802025190, 1.000000000000000000),
 ( 1.000000000000000000, 0.7024871511245815991, 1.000000000000000000),
 ( 1.000000000000000000, 0.7045189649009933053, 1.000000000000000000),
 ( 1.000000000000000000, 0.7054698226116191684, 1.000000000000000000),
 ( 1.000000000000000000, 0.7072451538296151696, 1.000000000000000000),
 ( 1.000000000000000000, 0.7080696632615188779, 1.000000000000000000),
 ( 1.000000000000000000, 0.7095909328304439434, 1.000000000000000000),
 ( 1.000000000000000000, 0.7102769625305951351, 1.000000000000000000),
 ( 1.000000000000000000, 0.7120402354171648796, 1.000000000000000000),
 ( 1.000000000000000000, 0.7128600990435562945, 1.000000000000000000),
 ( 1.000000000000000000, 0.7136629434598023014, 1.000000000000000000),
 ( 1.000000000000000000, 0.7138590768182416779, 1.000000000000000000),
 ( 1.000000000000000000, 0.7141136962395474574, 1.000000000000000000),
 ( 1.000000000000000000, 0.7141632686186834000, 1.000000000000000000),
 ( 1.000000000000000000, 0.7141258579405006524, 1.000000000000000000),
 ( 1.000000000000000000, 0.7138566471735118268, 1.000000000000000000),
 ( 1.000000000000000000, 0.7130110457638262345, 1.000000000000000000),
 ( 1.000000000000000000, 0.7124421886026640616, 1.000000000000000000),
 ( 1.000000000000000000, 0.7115151177449636766, 1.000000000000000000),
 ( 1.000000000000000000, 0.7111938932540499136, 1.000000000000000000),
 ( 1.000000000000000000, 0.7105477981655051734, 1.000000000000000000),
 ( 1.000000000000000000, 0.7102218485250791913, 1.000000000000000000),
 ( 1.000000000000000000, 0.7092850706994120458, 1.000000000000000000),
 ( 1.000000000000000000, 0.7087083600013776019, 1.000000000000000000),
 ( 1.000000000000000000, 0.7077862628354428809, 1.000000000000000000),
 ( 1.000000000000000000, 0.7074374214232334035, 1.000000000000000000),
 ( 1.000000000000000000, 0.7072571230115936025, 1.000000000000000000) ) ) 
 REPRESENTATION_ITEM ( '' )  SURFACE ( )  );
#12969=CARTESIAN_POINT ( 'NONE',  ( -222.0824530901772675, 149.3436370173336059, -5.265047855996057180 ) ) ;
#12983=CARTESIAN_POINT ( 'NONE',  ( -205.9652191273047777, 131.2378527988410326, 1.515400478619091329 ) ) ;
#12986=LINE ( 'NONE', #2177, #14603 ) ;
#12994=CARTESIAN_POINT ( 'NONE',  ( -224.1161033238799121, 145.7000333943786927, -3.784926783786191518 ) ) ;
#12995=CARTESIAN_POINT ( 'NONE',  ( -223.2420850427828327, 142.7740955428692757, 6.010832199141798782 ) ) ;
#13010=AXIS2_PLACEMENT_3D ( 'NONE', #12663, #3277, #4374 ) ;
#13028=EDGE_CURVE ( 'NONE', #3064, #1731, #13715, .T. ) ;
#13034=CARTESIAN_POINT ( 'NONE',  ( -188.3338018137096128, 131.5603057966125675, -5.230826428279604201 ) ) ;
#13048=CARTESIAN_POINT ( 'NONE',  ( -223.5674327266374917, 142.0998017908669624, 1.142491232282270008 ) ) ;
#13049=CARTESIAN_POINT ( 'NONE',  ( -225.7548303624725179, 142.7639966680278576, 3.410453015226076801 ) ) ;
#13057=CARTESIAN_POINT ( 'NONE',  ( -184.9746689684865260, 119.2870100535896682, 2.431555724346862846 ) ) ;
#13064=CARTESIAN_POINT ( 'NONE',  ( -223.1092991286456595, 142.9943895293494052, -1.544005151573194068 ) ) ;
#13067=CARTESIAN_POINT ( 'NONE',  ( -218.6461639067876206, 151.4790071514009639, 9.088489419225989963 ) ) ;
#13074=CARTESIAN_POINT ( 'NONE',  ( -193.7200834347810599, 142.0619459586758921, 2.500000000000000000 ) ) ;
#13097=CARTESIAN_POINT ( 'NONE',  ( -224.1564255670275827, 145.6277897662952228, 5.545703538890369266 ) ) ;
#13100=CARTESIAN_POINT ( 'NONE',  ( -218.1600191662880661, 152.2676192875508718, 2.431557144026069928 ) ) ;
#13116=CARTESIAN_POINT ( 'NONE',  ( -214.8715905313398480, 153.8675021612092451, 2.500000000000000000 ) ) ;
#13120=CARTESIAN_POINT ( 'NONE',  ( -193.9023367725753815, 141.7188637290702502, -0.4547266291960752049 ) ) ;
#13134=CARTESIAN_POINT ( 'NONE',  ( -201.1640730962011219, 128.1953734590158263, 3.478895870929496148 ) ) ;
#13137=CARTESIAN_POINT ( 'NONE',  ( -196.0016709267559349, 137.8086561579936813, 9.578254705571842109 ) ) ;
#13146=CARTESIAN_POINT ( 'NONE',  ( -224.3577192345715048, 145.2671405631149355, 0.1302923618042369780 ) ) ;
#13152=CARTESIAN_POINT ( 'NONE',  ( -187.9132138465967898, 138.8208849330412988, 2.500000000000000000 ) ) ;
#13167=CARTESIAN_POINT ( 'NONE',  ( -179.9267697467775520, 134.3633106217456543, 2.500000000000000000 ) ) ;
#13176=CARTESIAN_POINT ( 'NONE',  ( -222.9033204732309343, 147.8729242461827198, 9.743095389425892705 ) ) ;
#13183=DIRECTION ( 'NONE',  ( 0.4873681696970819655, 0.8731965799097684000, 0.000000000000000000 ) ) ;
#13193=CARTESIAN_POINT ( 'NONE',  ( -189.8662655649658859, 135.3588663075204579, -4.640918829492423292 ) ) ;
#13212=CARTESIAN_POINT ( 'NONE',  ( -179.1973253475678121, 117.8771479419235675, 5.305259944336949474 ) ) ;
#13215=CARTESIAN_POINT ( 'NONE',  ( -175.8063512637129975, 129.6626919947313468, 7.909502539118761888 ) ) ;
#13226=CARTESIAN_POINT ( 'NONE',  ( -220.7075610805327415, 147.6932589714580217, 9.903996657696321648 ) ) ;
#13230=CARTESIAN_POINT ( 'NONE',  ( -214.8715905313398480, 153.8675021612092451, 2.500000000000000000 ) ) ;
#13251=CARTESIAN_POINT ( 'NONE',  ( -224.0093084580825575, 145.8913731604616828, 8.788474005012725243 ) ) ;
#13252=ORIENTED_EDGE ( 'NONE', *, *, #9696, .T. ) ;
#13258=DIRECTION ( 'NONE',  ( 0.4873681696970831312, 0.8731965799097676229, 0.000000000000000000 ) ) ;
#13273=CARTESIAN_POINT ( 'NONE',  ( -207.1016862382755335, 146.9901175548950505, -2.963320117457100888 ) ) ;
#13281=( LENGTH_UNIT ( ) NAMED_UNIT ( * ) SI_UNIT ( .MILLI., .METRE. ) );
#13288=CARTESIAN_POINT ( 'NONE',  ( -209.4369489341841586, 132.9646294043573675, 3.478895870929508582 ) ) ;
#13292=CARTESIAN_POINT ( 'NONE',  ( -208.4664676862339832, 144.5514869593766036, 9.578254705571838556 ) ) ;
#13302=CARTESIAN_POINT ( 'NONE',  ( -223.5670544175258101, 142.1005145561789789, 1.135202858279962701 ) ) ;
#13313=( LENGTH_UNIT ( ) NAMED_UNIT ( * ) SI_UNIT ( .MILLI., .METRE. ) );
#13322=CARTESIAN_POINT ( 'NONE',  ( -198.5677679834141713, 144.7676449960911498, 2.500000000000000000 ) ) ;
#13330=CARTESIAN_POINT ( 'NONE',  ( -222.4858765390136455, 148.6208405819451173, 7.858754932069772714 ) ) ;
#13354=CARTESIAN_POINT ( 'NONE',  ( -179.6520503532206021, 128.8169225571170102, -4.640918829492417075 ) ) ;
#13372=CARTESIAN_POINT ( 'NONE',  ( -222.0824530901772675, 149.3436370173336059, -5.265047855996057180 ) ) ;
#13375=CARTESIAN_POINT ( 'NONE',  ( -187.1267843490969369, 133.7770572797440991, 9.578254705571838556 ) ) ;
#13381=VERTEX_POINT ( 'NONE', #8218 ) ;
#13382=CARTESIAN_POINT ( 'NONE',  ( -201.1639158238212417, 128.1956685377806764, 2.431555724346862402 ) ) ;
#13411=CARTESIAN_POINT ( 'NONE',  ( -219.8226924780726392, 153.3923528764989328, 5.388728173633870355 ) ) ;
#13414=CARTESIAN_POINT ( 'NONE',  ( -222.3134187894897309, 148.9298257115060551, 9.923566759394379488 ) ) ;
#13435=CARTESIAN_POINT ( 'NONE',  ( -174.7802519396333878, 131.5011100042426904, 1.515441477806783066 ) ) ;
#13448=CARTESIAN_POINT ( 'NONE',  ( -221.7276441040589248, 145.6842803271907201, -4.311380161871197991 ) ) ;
#13450=CARTESIAN_POINT ( 'NONE',  ( -186.4817914481332366, 122.8418524018552063, -2.964974570226826867 ) ) ;
#13453=CARTESIAN_POINT ( 'NONE',  ( -191.1905365997726562, 133.0085349363843363, 10.16010209732750624 ) ) ;
#13467=CARTESIAN_POINT ( 'NONE',  ( -201.8702151432138692, 146.6006509202294410, 3.478855109513426580 ) ) ;
#13479=CARTESIAN_POINT ( 'NONE',  ( -188.8176989649505231, 137.2180184133358694, 7.919662025281898998 ) ) ;
#13484=CARTESIAN_POINT ( 'NONE',  ( -219.6568521205180957, 153.6894819096027049, 4.764702133902800618 ) ) ;
#13486=CARTESIAN_POINT ( 'NONE',  ( -217.2009144557466129, 154.0222411784483825, 6.228828271822901996 ) ) ;
#13522=CARTESIAN_POINT ( 'NONE',  ( -217.3713917269321598, 153.7233570374494320, -1.908609582020496021 ) ) ;
#13523=CARTESIAN_POINT ( 'NONE',  ( -171.9831566630682858, 119.3897064310878875, -4.822481523602708542 ) ) ;
#13526=CARTESIAN_POINT ( 'NONE',  ( -225.5658467874630446, 143.1025904080742919, 5.367833425961707761 ) ) ;
#13536=CARTESIAN_POINT ( 'NONE',  ( -174.7889847475609599, 131.4854638080208247, 3.478855109783925315 ) ) ;
#13552=CARTESIAN_POINT ( 'NONE',  ( -172.5511497006709192, 129.7930440361603246, 5.430596897033706405 ) ) ;
#13559=CARTESIAN_POINT ( 'NONE',  ( -224.1569016198369297, 145.6269368429599638, 5.559760092157292277 ) ) ;
#13561=CARTESIAN_POINT ( 'NONE',  ( -222.1447695234329842, 149.2319873451267824, 7.942449175544537887 ) ) ;
#13599=CARTESIAN_POINT ( 'NONE',  ( -222.6001360064667267, 143.9905737129706438, -2.961424432328688461 ) ) ;
#13601=CARTESIAN_POINT ( 'NONE',  ( -173.0624365063895311, 117.4516868700737433, -3.188270265946634208 ) ) ;
#13606=CARTESIAN_POINT ( 'NONE',  ( -184.7761983179757976, 119.6423109536379883, 5.434137442415926778 ) ) ;
#13618=CARTESIAN_POINT ( 'NONE',  ( -193.9262940755599232, 141.6759404601118320, 5.434754235172606585 ) ) ;
#13633=CARTESIAN_POINT ( 'NONE',  ( -218.6367072074390592, 155.5172316571506599, -0.02616420791762594927 ) ) ;
#13634=CARTESIAN_POINT ( 'NONE',  ( -193.9262940755599232, 141.6759404601118320, 5.434754235172606585 ) ) ;
#13639=CARTESIAN_POINT ( 'NONE',  ( -222.9820152130263295, 147.7319302668168177, 7.565779686223725875 ) ) ;
#13641=CARTESIAN_POINT ( 'NONE',  ( -219.1834294040782538, 150.5104683866151731, 9.570045470580922142 ) ) ;
#13643=CARTESIAN_POINT ( 'NONE',  ( -168.5715549668454685, 126.2102699412402700, -2.485716223453637852 ) ) ;
#13652=SHAPE_REPRESENTATION ( 'Handle Grip', ( #12337 ), #4745 ) ;
#13673=LINE ( 'NONE', #2878, #9477 ) ;
#13681=CARTESIAN_POINT ( 'NONE',  ( -220.4755021374134287, 148.0753638217371702, -5.053461931965367526 ) ) ;
#13682=CARTESIAN_POINT ( 'NONE',  ( -187.3343951027933656, 121.3449523462597313, -0.4555467707853332882 ) ) ;
#13685=CARTESIAN_POINT ( 'NONE',  ( -213.9961813491638623, 134.6717504882919911, 3.478895870929492595 ) ) ;
#13701=CARTESIAN_POINT ( 'NONE',  ( -207.0940556909077657, 149.0079180481279479, 5.434754235172608361 ) ) ;
#13715=B_SPLINE_CURVE_WITH_KNOTS ( 'NONE', 3,
 ( #5746, #12923, #10560, #14488, #8217, #11986, #14414, #7258, #4878, #14331, #3534, #15513, #2112, #13067, #7099, #1155, #5981, #3455, #2349, #5823, #8367, #13226, #15590, #9619, #4558, #10643, #8446, #7184, #15435, #10885, #2426, #8287, #2268, #9384, #12053, #12995, #6069, #11904, #1079, #2187, #9699, #10720, #6944, #11751 ),
 .UNSPECIFIED., .F., .F.,
 ( 4, 2, 2, 2, 2, 2, 2, 2, 2, 2, 2, 2, 2, 2, 2, 2, 2, 2, 2, 2, 2, 4 ),
 ( 0.02425151066300419017, 0.02566658695633274381, 0.02708166324966130092, 0.02778920139632557254, 0.02849673954298984069, 0.02991181583631835617, 0.03132689212964687164, 0.03203443027631112938, 0.03274196842297538712, 0.03415704471630390260, 0.03557212100963242501, 0.03698719730296094743, 0.03769473544962523986, 0.03840227359628953230, 0.03981734988961815880, 0.04123242618294678530, 0.04193996432961112630, 0.04264750247627546037, 0.04406257876960419095, 0.04477011691626857359, 0.04547765506293295623, 0.04689273135626172151 ),
 .UNSPECIFIED. ) ;
#13722=CARTESIAN_POINT ( 'NONE',  ( -223.8893703921771419, 146.1062610326309823, -1.348932811884229421 ) ) ;
#13725=CARTESIAN_POINT ( 'NONE',  ( -217.2630589882568870, 153.9147002545655027, 6.438236223713596829 ) ) ;
#13727=CARTESIAN_POINT ( 'NONE',  ( -170.7457446375415770, 122.3148678559813476, -5.128095649471044126 ) ) ;
#13744=CARTESIAN_POINT ( 'NONE',  ( -185.2055264765504887, 137.3096093875189467, 2.500000000000000000 ) ) ;
#13763=CARTESIAN_POINT ( 'NONE',  ( -167.6561596704311512, 127.1594819807359329, -0.4629209656553701646 ) ) ;
#13766=CARTESIAN_POINT ( 'NONE',  ( -176.6594047394515314, 116.7136007993067324, 1.317773660835219740 ) ) ;
#13779=CARTESIAN_POINT ( 'NONE',  ( -219.6650276661029011, 145.2909210783078890, 9.577123744044234499 ) ) ;
#13789=DIRECTION ( 'NONE',  ( 0.4873681696970831312, 0.8731965799097676229, 0.000000000000000000 ) ) ;
#13791=CARTESIAN_POINT ( 'NONE',  ( -218.7216426999998191, 155.3650563895502046, -0.4850387387758420266 ) ) ;
#13800=CARTESIAN_POINT ( 'NONE',  ( -220.5194744645034746, 152.1439585714864791, 6.950724492665587562 ) ) ;
#13823=CARTESIAN_POINT ( 'NONE',  ( -218.4444600228138711, 155.8616726660956715, 2.500000000270498735 ) ) ;
#13826=DIRECTION ( 'NONE',  ( 0.000000000000000000, -0.9953154669545954958, -0.09668051117446378739 ) ) ;
#13842=CARTESIAN_POINT ( 'NONE',  ( -185.3517468524019591, 137.0386009272039871, -0.4547266291960738172 ) ) ;
#13845=CARTESIAN_POINT ( 'NONE',  ( -225.5636091402884915, 143.1065995042388863, -0.5218507872395625746 ) ) ;
#13865=CARTESIAN_POINT ( 'NONE',  ( -174.6331699355062028, 120.3494046152724763, 9.441255307061881652 ) ) ;
#13877=CARTESIAN_POINT ( 'NONE',  ( -174.1990073215050643, 116.1278056868591904, 4.018260756276598400 ) ) ;
#13885=CARTESIAN_POINT ( 'NONE',  ( -222.8948771076028947, 147.8880518610581305, -2.733432078552652023 ) ) ;
#13889=CARTESIAN_POINT ( 'NONE',  ( -174.2806066667207858, 115.9816076509688401, 1.710173242044437991 ) ) ;
#13925=CARTESIAN_POINT ( 'NONE',  ( -193.7157043470890301, 142.0697917816768836, 1.515441477536284332 ) ) ;
#13928=CARTESIAN_POINT ( 'NONE',  ( -179.1950877003932874, 117.8811570380880909, -0.5844242688643165318 ) ) ;
#13941=CARTESIAN_POINT ( 'NONE',  ( -223.5464781713420734, 146.7206062712571111, 9.530069280832668355 ) ) ;
#13953=CARTESIAN_POINT ( 'NONE',  ( -173.8627125986912176, 116.7303304721469885, 5.982824555829307833 ) ) ;
#13954=CARTESIAN_POINT ( 'NONE',  ( -219.3428653954115646, 154.2520384152134625, -2.513716752921474118 ) ) ;
#13964=CARTESIAN_POINT ( 'NONE',  ( -220.8828325426286767, 151.4929455369283176, -2.526440127944020286 ) ) ;
#13992=DIRECTION ( 'NONE',  ( 0.8731965799097682890, -0.4873681696970819099, -0.000000000000000000 ) ) ;
#13997=CARTESIAN_POINT ( 'NONE',  ( -198.7485669925355012, 144.4350871509360559, -0.4547266291960735951 ) ) ;
#14001=CARTESIAN_POINT ( 'NONE',  ( -173.2784152866543934, 122.7799518889917465, -5.329639836781006501 ) ) ;
#14012=CARTESIAN_POINT ( 'NONE',  ( -190.6501653245252044, 127.3085702864440520, 7.918248976830637886 ) ) ;
#14025=CARTESIAN_POINT ( 'NONE',  ( -223.7640232666028623, 146.3308400842772130, -1.599190326327902367 ) ) ;
#14033=CARTESIAN_POINT ( 'NONE',  ( -224.3206423883182765, 145.3335695532608440, -0.03206942370135386355 ) ) ;
#14052=CARTESIAN_POINT ( 'NONE',  ( -223.5992072901615018, 142.0487386537765246, 3.276137811062253213 ) ) ;
#14072=CARTESIAN_POINT ( 'NONE',  ( -212.2154691228631691, 150.1790628786027355, -2.963320117457098224 ) ) ;
#14075=CARTESIAN_POINT ( 'NONE',  ( -199.2233958860587961, 127.9753750774359276, -0.4555467707853375070 ) ) ;
#14087=CARTESIAN_POINT ( 'NONE',  ( -187.1267843490969369, 133.7770572797440991, 9.578254705571838556 ) ) ;
#14099=CARTESIAN_POINT ( 'NONE',  ( -174.2675151123989110, 116.0050632255638163, 3.108104069861567620 ) ) ;
#14101=CARTESIAN_POINT ( 'NONE',  ( -220.0780021574012721, 148.8225603397216901, -5.061978238651692941 ) ) ;
#14154=CARTESIAN_POINT ( 'NONE',  ( -186.4817914481332366, 122.8418524018552063, -2.964974570226826867 ) ) ;
#14167=CARTESIAN_POINT ( 'NONE',  ( -179.3772030532177837, 117.5545944912402661, 3.345861034185851235 ) ) ;
#14178=CARTESIAN_POINT ( 'NONE',  ( -222.4732244369151886, 144.2379617518073474, -3.208335888254660428 ) ) ;
#14225=DIRECTION ( 'NONE',  ( 0.05375305303998870188, 0.09630703232712070627, -0.9938991723576509063 ) ) ;
#14228=CARTESIAN_POINT ( 'NONE',  ( -208.3893201713671033, 134.8533518211819739, -2.964974570226836192 ) ) ;
#14243=CARTESIAN_POINT ( 'NONE',  ( -223.5918188539070002, 142.0538562971642307, 1.612306317632525854 ) ) ;
#14244=CARTESIAN_POINT ( 'NONE',  ( -184.9748306402843809, 119.2867206268225999, 3.478895870929497036 ) ) ;
#14258=CARTESIAN_POINT ( 'NONE',  ( -220.3095741282960773, 148.3879606264429754, -5.070227393135747107 ) ) ;
#14297=CARTESIAN_POINT ( 'NONE',  ( -206.8718859864436581, 149.4025266312245037, 2.500000000000000000 ) ) ;
#14300=CARTESIAN_POINT ( 'NONE',  ( -194.3489852843322581, 137.1051365066642234, -4.640918829492427733 ) ) ;
#14317=CARTESIAN_POINT ( 'NONE',  ( -199.4124801547868913, 127.6177204676982910, 3.478895870929493483 ) ) ;
#14330=CARTESIAN_POINT ( 'NONE',  ( -223.9140261897964876, 146.0620863009135348, -4.050555112215771913 ) ) ;
#14331=CARTESIAN_POINT ( 'NONE',  ( -217.6520716543167282, 153.2380971607960589, 7.506281845139713305 ) ) ;
#14363=CARTESIAN_POINT ( 'NONE',  ( -223.3687964238177983, 147.0389510131371367, 9.463477258803484560 ) ) ;
#14384=CARTESIAN_POINT ( 'NONE',  ( -174.9627087613145306, 131.1742099673107305, -0.4568654681747568169 ) ) ;
#14399=CARTESIAN_POINT ( 'NONE',  ( -194.4337897068680547, 127.2572260587109554, 3.478895870929501033 ) ) ;
#14402=CARTESIAN_POINT ( 'NONE',  ( -213.3956520262682091, 148.0073597223720583, 9.578254705571842109 ) ) ;
#14414=CARTESIAN_POINT ( 'NONE',  ( -217.2422530631390600, 153.9507230298087848, 6.369419626229976927 ) ) ;
#14430=AXIS2_PLACEMENT_3D ( 'NONE', #10759, #11941, #13183 ) ;
#14440=CARTESIAN_POINT ( 'NONE',  ( -223.2365180022060542, 142.7849184768047337, 6.010681374827787415 ) ) ;
#14461=CARTESIAN_POINT ( 'NONE',  ( -172.5271923976867470, 129.8359673051191123, -0.4588839673349612291 ) ) ;
#14472=VERTEX_POINT ( 'NONE', #1629 ) ;
#14475=CARTESIAN_POINT ( 'NONE',  ( -213.7840885461983760, 135.0504928752735339, -0.4555467707853347870 ) ) ;
#14478=CARTESIAN_POINT ( 'NONE',  ( -177.2599095556795419, 121.3508012008377932, 9.485662293947264345 ) ) ;
#14488=CARTESIAN_POINT ( 'NONE',  ( -216.9323607303195729, 154.4852837081892574, 5.108206056088243407 ) ) ;
#14505=CARTESIAN_POINT ( 'NONE',  ( -206.8762397066792005, 149.3947262580036863, 3.478855109513426580 ) ) ;
#14514=CARTESIAN_POINT ( 'NONE',  ( -224.5769159865018594, 144.8744151739456925, 3.251642181181148672 ) ) ;
#14516=CARTESIAN_POINT ( 'NONE',  ( -221.1308609718745117, 146.8914367518880226, 9.717582667742421521 ) ) ;
#14536=CARTESIAN_POINT ( 'NONE',  ( -193.1449676018668526, 139.3614456044060148, -2.963320117457103109 ) ) ;
#14549=CARTESIAN_POINT ( 'NONE',  ( -200.1353104204616500, 130.1171604195963880, -2.964974570226841522 ) ) ;
#14551=CARTESIAN_POINT ( 'NONE',  ( -220.8021227237918254, 143.2564083082033619, 7.918248976830615682 ) ) ;
#14554=VERTEX_POINT ( 'NONE', #4622 ) ;
#14561=CARTESIAN_POINT ( 'NONE',  ( -223.3090784427782864, 142.6032858358233000, -0.6846340373356000208 ) ) ;
#14567=CARTESIAN_POINT ( 'NONE',  ( -185.2055264765504887, 137.3096093875189467, 2.500000000000000000 ) ) ;
#14578=DIRECTION ( 'NONE',  ( 0.8731965799097682890, -0.4873681696970819099, 0.000000000000000000 ) ) ;
#14590=CARTESIAN_POINT ( 'NONE',  ( -220.6606568355639411, 151.8910081918378125, 7.146912864506841601 ) ) ;
#14593=CARTESIAN_POINT ( 'NONE',  ( -223.4360080598686693, 146.9185308168432584, 7.053220276998304783 ) ) ;
#14598=AXIS2_PLACEMENT_3D ( 'NONE', #9488, #3244, #11538 ) ;
#14603=VECTOR ( 'NONE', #12911, 1000.000000000000114 ) ;
#14618=CARTESIAN_POINT ( 'NONE',  ( -209.2730951545231335, 145.1348166524657302, -4.640918829492436615 ) ) ;
#14622=CIRCLE ( 'NONE', #1007, 4.499999999999950262 ) ;
#14636=CARTESIAN_POINT ( 'NONE',  ( -217.0245320789650805, 154.3266673407848941, -0.6962477592939494420 ) ) ;
#14637=CARTESIAN_POINT ( 'NONE',  ( -185.2102393155530535, 125.0770951282925409, -4.642206099734998759 ) ) ;
#14640=CARTESIAN_POINT ( 'NONE',  ( -208.4006302466032992, 134.8330880460140122, 7.918248976830637886 ) ) ;
#14648=CARTESIAN_POINT ( 'NONE',  ( -223.2622533207028539, 142.6949529005080421, -0.9050894319243404373 ) ) ;
#14652=CARTESIAN_POINT ( 'NONE',  ( -193.1820620331849341, 139.2949851078578831, 7.919662025281897222 ) ) ;
#14666=CARTESIAN_POINT ( 'NONE',  ( -177.5673841713239085, 132.5493133318365437, 5.434754235172600367 ) ) ;
#14670=CARTESIAN_POINT ( 'NONE',  ( -219.5914105103326790, 153.8067308268499858, 4.439047251926309556 ) ) ;
#14672=CARTESIAN_POINT ( 'NONE',  ( -221.5674180155096167, 146.0573998878414841, 9.414961245066379547 ) ) ;
#14674=CARTESIAN_POINT ( 'NONE',  ( -173.6511438682215953, 117.1093890634716672, -2.227947778868676565 ) ) ;
#14708=CARTESIAN_POINT ( 'NONE',  ( -216.0630845075784805, 143.0974466248333954, -4.642206099735013858 ) ) ;
#14713=CARTESIAN_POINT ( 'NONE',  ( -200.1466204956978459, 130.0968966444285968, 7.918248976830634334 ) ) ;
#14727=CARTESIAN_POINT ( 'NONE',  ( -214.8759442515754188, 153.8597017879883424, 3.478855109513426580 ) ) ;
#14732=ORIENTED_EDGE ( 'NONE', *, *, #137, .T. ) ;
#14741=CARTESIAN_POINT ( 'NONE',  ( -174.7889847475609599, 131.4854638080208247, 3.478855109783925315 ) ) ;
#14745=CARTESIAN_POINT ( 'NONE',  ( -223.1382750711026404, 147.4519662024128479, 7.419826817990093026 ) ) ;
#14747=CARTESIAN_POINT ( 'NONE',  ( -219.5899114050779417, 153.8094167092946520, 7.921877796732283095 ) ) ;
#14749=CARTESIAN_POINT ( 'NONE',  ( -169.8738088132719213, 123.8770777559960692, -4.653609069845229484 ) ) ;
#14780=CARTESIAN_POINT ( 'NONE',  ( -219.8172205651076752, 149.3079862779945302, -4.999365138195623892 ) ) ;
#14781=CARTESIAN_POINT ( 'NONE',  ( -193.5420962672365022, 128.8371742780315969, -2.964974570226833084 ) ) ;
#14783=CARTESIAN_POINT ( 'NONE',  ( -209.2398179475638926, 133.3202902034983595, 5.434137442415948094 ) ) ;
#14796=CARTESIAN_POINT ( 'NONE',  ( -179.9311234670130943, 134.3555102485248369, 3.478855109513426580 ) ) ;
#14810=CARTESIAN_POINT ( 'NONE',  ( -198.7725242955204692, 144.3921638819772113, 5.434754235172606585 ) ) ;
#14817=CARTESIAN_POINT ( 'NONE',  ( -222.6528199517674125, 148.3217352523010959, 7.791448390692321979 ) ) ;
#14819=CARTESIAN_POINT ( 'NONE',  ( -221.4570519113204341, 150.4641414006810294, 7.827120672804973367 ) ) ;
#14861=CARTESIAN_POINT ( 'NONE',  ( -219.6417540138374704, 145.3326194796887023, -4.642206099735023628 ) ) ;
#14864=CARTESIAN_POINT ( 'NONE',  ( -190.6501653245252044, 127.3085702864440520, 7.918248976830637886 ) ) ;
#14868=CARTESIAN_POINT ( 'NONE',  ( -216.7216729069047005, 154.8463875879168086, 3.280095325655492111 ) ) ;
#14876=VERTEX_POINT ( 'NONE', #10149 ) ;
#14878=CARTESIAN_POINT ( 'NONE',  ( -174.9866660642990155, 131.1312866983521701, 5.432615396193912538 ) ) ;
#14893=CARTESIAN_POINT ( 'NONE',  ( -220.1893657699912694, 152.7354001160292682, -1.484330510404517911 ) ) ;
#14902=CARTESIAN_POINT ( 'NONE',  ( -221.2092521592557546, 150.9081135545043821, 7.674399710142353115 ) ) ;
#14906=CARTESIAN_POINT ( 'NONE',  ( -168.1636048451761951, 126.9411766215776396, -1.100011624693940870 ) ) ;
#14941=CARTESIAN_POINT ( 'NONE',  ( -193.1449676018668526, 139.3614456044060148, -2.963320117457103109 ) ) ;
#14944=CARTESIAN_POINT ( 'NONE',  ( -201.1640730962011219, 128.1953734590158263, 1.515400478619091773 ) ) ;
#14955=CARTESIAN_POINT ( 'NONE',  ( -207.9892458934089632, 147.4169567187306029, 7.919662025281897222 ) ) ;
#14966=CARTESIAN_POINT ( 'NONE',  ( -219.2661329852160748, 154.3895165730399412, -2.326617110117079612 ) ) ;
#14977=CARTESIAN_POINT ( 'NONE',  ( -219.0707735969879195, 150.7146073354513476, 9.486927387000964274 ) ) ;
#14979=CARTESIAN_POINT ( 'NONE',  ( -167.9381859705957254, 127.3450499201829160, 0.2100378832225609782 ) ) ;
#14987=EDGE_LOOP ( 'NONE', ( #15393, #8975, #4825, #9177 ) ) ;
#15002=CARTESIAN_POINT ( 'NONE',  ( -169.9318100387881714, 128.7846982781319412, 2.500000000781056997 ) ) ;
#15018=CARTESIAN_POINT ( 'NONE',  ( -188.7806045336324132, 137.2844789098840863, -2.963320117457101777 ) ) ;
#15021=CARTESIAN_POINT ( 'NONE',  ( -218.1518098834511648, 139.2461763302102327, 1.515400478619101987 ) ) ;
#15032=CARTESIAN_POINT ( 'NONE',  ( -182.2596580518439850, 130.2653702959948987, 9.578254705571840333 ) ) ;
#15043=CARTESIAN_POINT ( 'NONE',  ( -168.5655597009508426, 126.2210114011889033, 7.273861828271574126 ) ) ;
#15044=CARTESIAN_POINT ( 'NONE',  ( -220.4547830239155246, 152.2598634421184727, -4.296684159728658692 ) ) ;
#15051=CARTESIAN_POINT ( 'NONE',  ( -219.4169439222603160, 154.1193151060158471, 2.705939130397310599 ) ) ;
#15065=EDGE_LOOP ( 'NONE', ( #189, #1451, #12512, #4838, #9564 ) ) ;
#15092=CARTESIAN_POINT ( 'NONE',  ( -206.2168697392640695, 148.5706983463157940, -0.4547266291960757045 ) ) ;
#15095=CARTESIAN_POINT ( 'NONE',  ( -221.5581585947747101, 141.9038310245542505, 5.434137442415940988 ) ) ;
#15111=CARTESIAN_POINT ( 'NONE',  ( -179.6920193139674780, 128.7453118898713456, 9.578254705571842109 ) ) ;
#15124=CARTESIAN_POINT ( 'NONE',  ( -168.3730750733982973, 126.5658778264387507, 6.698921820633309210 ) ) ;
#15125=CARTESIAN_POINT ( 'NONE',  ( -219.4139989654581768, 154.1245914584070533, 2.346545549012409637 ) ) ;
#15134=CARTESIAN_POINT ( 'NONE',  ( -219.4360840196855804, 154.0850226169901305, 3.058976617611859794 ) ) ;
#15153=CARTESIAN_POINT ( 'NONE',  ( -224.6032697205328645, 144.8271983225910162, 2.539373236809186807 ) ) ;
#15170=CARTESIAN_POINT ( 'NONE',  ( -206.8675068987516283, 149.4103724542255804, 1.515441477536285220 ) ) ;
#15173=CARTESIAN_POINT ( 'NONE',  ( -173.0624365063895311, 117.4516868700737433, -3.188270265946634208 ) ) ;
#15189=CARTESIAN_POINT ( 'NONE',  ( -220.8021227237918254, 143.2564083082033619, 7.918248976830615682 ) ) ;
#15201=CARTESIAN_POINT ( 'NONE',  ( -168.8600800343791377, 125.6933319919581464, 7.985209213891318214 ) ) ;
#15202=CARTESIAN_POINT ( 'NONE',  ( -222.5547230352208032, 144.0789707147005458, -3.043139129519528030 ) ) ;
#15211=CARTESIAN_POINT ( 'NONE',  ( -224.1994838848473250, 145.5506440309058860, -0.5027386702675625818 ) ) ;
#15219=CARTESIAN_POINT ( 'NONE',  ( -206.8718859864436581, 149.4025266312245037, 2.500000000000000000 ) ) ;
#15245=CARTESIAN_POINT ( 'NONE',  ( -211.4625087271040513, 151.5689812133889234, -0.4547266291960755935 ) ) ;
#15249=CARTESIAN_POINT ( 'NONE',  ( -210.8320337336493822, 142.3623933791497791, -5.230826428279598872 ) ) ;
#15262=CARTESIAN_POINT ( 'NONE',  ( -170.8670245162619779, 127.1065088405712373, 7.890326795182211583 ) ) ;
#15275=CARTESIAN_POINT ( 'NONE',  ( -172.3086228175700398, 119.5147262659699265, 9.219235224006146368 ) ) ;
#15276=CARTESIAN_POINT ( 'NONE',  ( -223.8857310410845969, 146.1127815013952898, -1.344505601181561927 ) ) ;
#15311=FACE_OUTER_BOUND ( 'NONE', #7448, .T. ) ;
#15326=CARTESIAN_POINT ( 'NONE',  ( -179.8633755235878198, 122.3938961877832696, -4.689260562946571120 ) ) ;
#15340=CARTESIAN_POINT ( 'NONE',  ( -224.7572118800429735, 144.5513867789856022, 7.859965607560822853 ) ) ;
#15351=CARTESIAN_POINT ( 'NONE',  ( -171.6707776135659174, 120.6575260737504180, 9.685254691063745369 ) ) ;
#15352=CARTESIAN_POINT ( 'NONE',  ( -221.8281913388289013, 149.7991868573274985, -5.066262527848913955 ) ) ;
#15369=CARTESIAN_POINT ( 'NONE',  ( -174.1824175338263387, 116.1575288956428409, 0.3248046258198108993 ) ) ;
#15393=ORIENTED_EDGE ( 'NONE', *, *, #3533, .F. ) ;
#15403=CARTESIAN_POINT ( 'NONE',  ( -179.9267697467775520, 134.3633106217456543, 2.500000000000000000 ) ) ;
#15406=CARTESIAN_POINT ( 'NONE',  ( -214.7080733591933779, 145.5905563435376848, -5.230826428279589990 ) ) ;
#15421=CARTESIAN_POINT ( 'NONE',  ( -218.1518098834511648, 139.2461763302102327, 1.515400478619101987 ) ) ;
#15433=CARTESIAN_POINT ( 'NONE',  ( -219.6164868915797967, 149.6803330067249931, -4.932213728819581533 ) ) ;
#15435=CARTESIAN_POINT ( 'NONE',  ( -222.1184893299650298, 144.9908166140801882, 8.775148900260887785 ) ) ;
#15448=CARTESIAN_POINT ( 'NONE',  ( -174.7846310273254176, 131.4932641812416421, 2.500000000270498735 ) ) ;
#15471=PLANE ( 'NONE',  #11553 ) ;
#15484=CARTESIAN_POINT ( 'NONE',  ( -199.5653198453618700, 142.9393910578133102, -2.963320117457100000 ) ) ;
#15495=FILL_AREA_STYLE_COLOUR ( '', #10152 ) ;
#15499=CARTESIAN_POINT ( 'NONE',  ( -183.9313806081839289, 121.1548445249323720, 7.918248976830652097 ) ) ;
#15507=CARTESIAN_POINT ( 'NONE',  ( -223.6145774380523505, 142.0129443944823606, 2.393984899497048513 ) ) ;
#15512=CARTESIAN_POINT ( 'NONE',  ( -222.3080144202387203, 148.9395084873732742, -3.019567288340968769 ) ) ;
#15513=CARTESIAN_POINT ( 'NONE',  ( -218.1626881431459992, 152.3400484335867304, 8.464914971617218953 ) ) ;
#15517=FACE_OUTER_BOUND ( 'NONE', #15065, .T. ) ;
#15534=CARTESIAN_POINT ( 'NONE',  ( -223.8367800313764064, 146.2004849192998961, 6.377934699871589785 ) ) ;
#15552=CARTESIAN_POINT ( 'NONE',  ( -193.7200834347810599, 142.0619459586758921, 2.500000000000000000 ) ) ;
#15556=CARTESIAN_POINT ( 'NONE',  ( -194.7245433579248868, 140.1837011942588447, -2.963320117457102665 ) ) ;
#15573=CARTESIAN_POINT ( 'NONE',  ( -194.2694872093395873, 127.5478817636406035, 5.434137442415935659 ) ) ;
#15576=ADVANCED_FACE ( 'NONE', ( #8241 ), #10440, .F. ) ;
#15578=CARTESIAN_POINT ( 'NONE',  ( -207.1471226269450767, 137.0919095985319132, 9.577123744044238052 ) ) ;
#15590=CARTESIAN_POINT ( 'NONE',  ( -220.9230348769640102, 147.2864796216551326, 9.830311889130468828 ) ) ;
#15604=ADVANCED_FACE ( 'NONE', ( #2215 ), #12966, .T. ) ;
ENDSEC;
END-ISO-10303-21;
